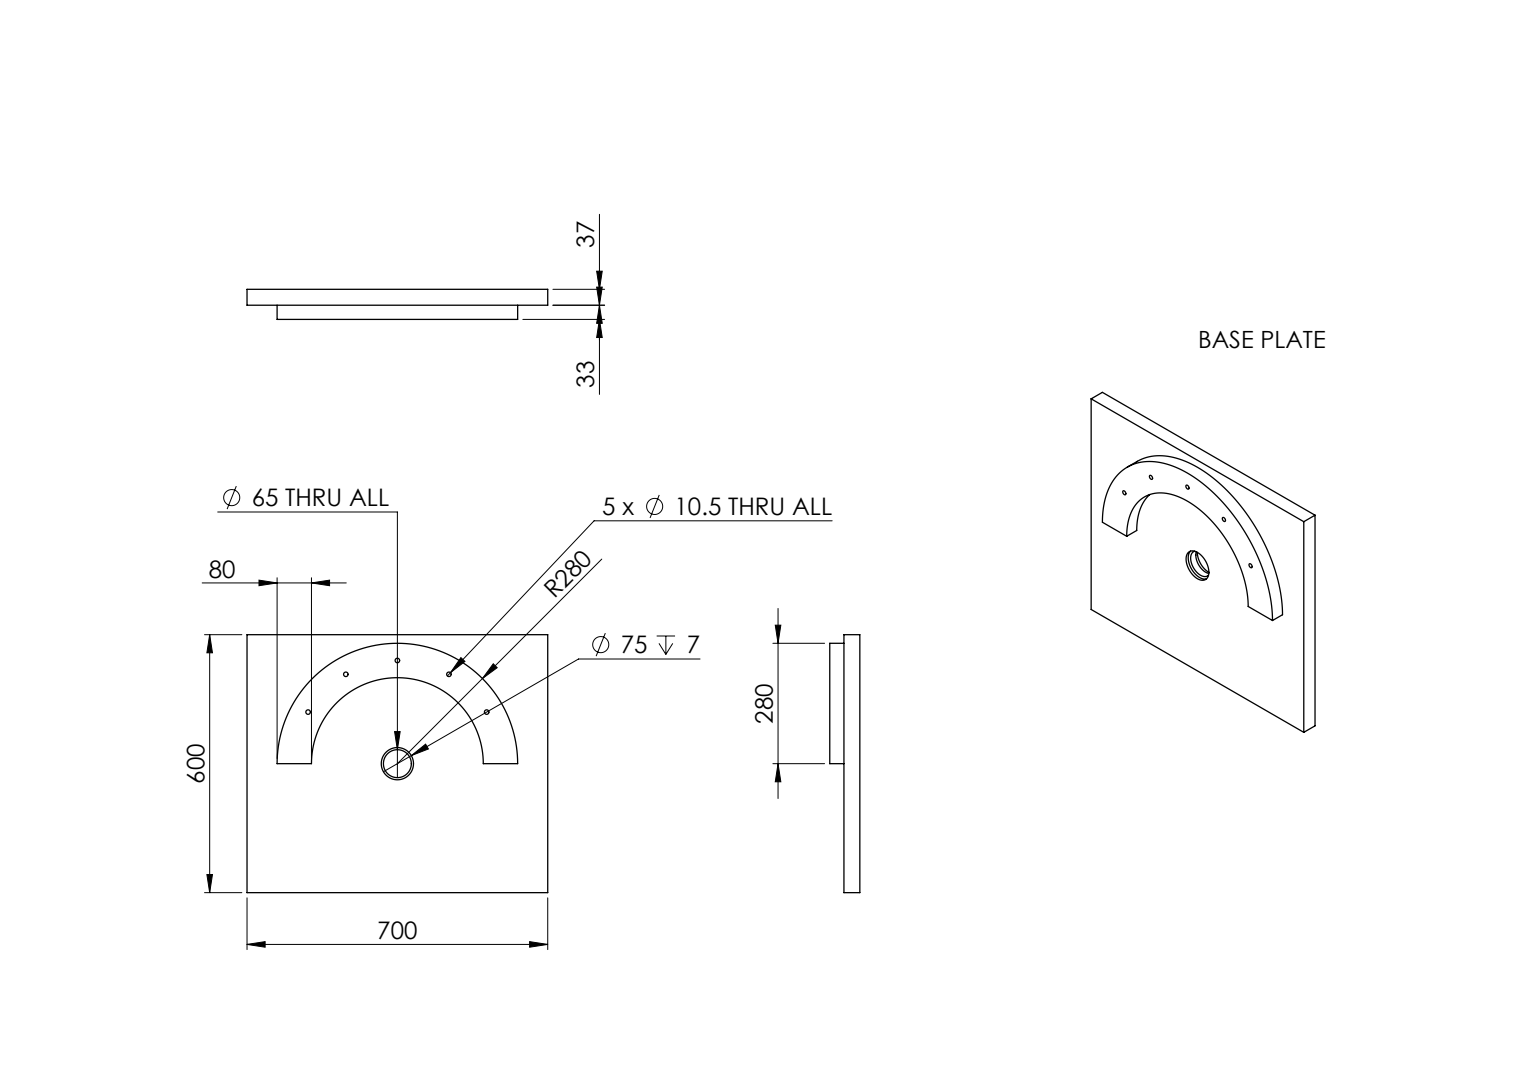
ISO-10303-21;
HEADER;
FILE_DESCRIPTION (('STEP AP214'),
    '1' );
FILE_NAME ('base plate.step',
    '2026-10-23T05:12:30',
    ( '' ),
    ( '' ),
    'SwSTEP 2.0',
    'SolidWorks 2026',
    '' );
FILE_SCHEMA (( 'AUTOMOTIVE_DESIGN' ));
ENDSEC;

DATA;
#3=SURFACE_STYLE_USAGE ( .BOTH. , #3079 ) ;
#17=DIRECTION ( 'NONE',  ( 1.000000000000000000, 0.000000000000000000, 0.000000000000000000 ) ) ;
#19=FACE_OUTER_BOUND ( 'NONE', #6377, .T. ) ;
#26=DIRECTION ( 'NONE',  ( -0.000000000000000000, -0.000000000000000000, 1.000000000000000000 ) ) ;
#42=ORIENTED_EDGE ( 'NONE', *, *, #2330, .T. ) ;
#45=AXIS2_PLACEMENT_3D ( 'NONE', #3946, #5204, #2688 ) ;
#49=ORIENTED_EDGE ( 'NONE', *, *, #2998, .F. ) ;
#51=DIRECTION ( 'NONE',  ( -0.000000000000000000, -0.000000000000000000, 1.000000000000000000 ) ) ;
#61=MECHANICAL_DESIGN_GEOMETRIC_PRESENTATION_REPRESENTATION('',(#4091),#6487);
#62=FACE_BOUND ( 'NONE', #7747, .T. ) ;
#67=DIRECTION ( 'NONE',  ( -0.000000000000000000, 0.000000000000000000, 1.000000000000000000 ) ) ;
#76=SURFACE_STYLE_FILL_AREA ( #5998 ) ;
#98=AXIS2_PLACEMENT_3D ( 'NONE', #4234, #3767, #1954 ) ;
#99=DIRECTION ( 'NONE',  ( 0.000000000000000000, 0.000000000000000000, 1.000000000000000000 ) ) ;
#107=ORIENTED_EDGE ( 'NONE', *, *, #1973, .T. ) ;
#109=ORIENTED_EDGE ( 'NONE', *, *, #3940, .F. ) ;
#123=DIRECTION ( 'NONE',  ( 1.000000000000000000, 0.000000000000000000, 0.000000000000000000 ) ) ;
#128=EDGE_CURVE ( 'NONE', #1948, #4169, #2830, .T. ) ;
#130=ORIENTED_EDGE ( 'NONE', *, *, #1178, .T. ) ;
#144=FACE_OUTER_BOUND ( 'NONE', #3867, .T. ) ;
#154=VERTEX_POINT ( 'NONE', #7084 ) ;
#160=DIRECTION ( 'NONE',  ( 1.000000000000000000, 0.000000000000000000, 0.000000000000000000 ) ) ;
#166=DIRECTION ( 'NONE',  ( -1.000000000000000000, 0.000000000000000000, 0.000000000000000000 ) ) ;
#182=FACE_OUTER_BOUND ( 'NONE', #3425, .T. ) ;
#185=VERTEX_POINT ( 'NONE', #2518 ) ;
#206=EDGE_LOOP ( 'NONE', ( #7630, #2753 ) ) ;
#208=FACE_OUTER_BOUND ( 'NONE', #6661, .T. ) ;
#217=ORIENTED_EDGE ( 'NONE', *, *, #263, .T. ) ;
#218=EDGE_CURVE ( 'NONE', #491, #1814, #4911, .T. ) ;
#245=CARTESIAN_POINT ( 'NONE',  ( 207.8429183184021269, 119.9981648402868331, -50.00000000000000000 ) ) ;
#253=FACE_OUTER_BOUND ( 'NONE', #5709, .T. ) ;
#257=VERTEX_POINT ( 'NONE', #4355 ) ;
#263=EDGE_CURVE ( 'NONE', #257, #1814, #3618, .T. ) ;
#265=ORIENTED_EDGE ( 'NONE', *, *, #789, .F. ) ;
#269=FACE_OUTER_BOUND ( 'NONE', #4910, .T. ) ;
#275=LINE ( 'NONE', #5724, #2339 ) ;
#329=LINE ( 'NONE', #3997, #6288 ) ;
#335=ORIENTED_EDGE ( 'NONE', *, *, #1569, .F. ) ;
#366=DIRECTION ( 'NONE',  ( 1.000000000000000000, 0.000000000000000000, 0.000000000000000000 ) ) ;
#376=LINE ( 'NONE', #524, #671 ) ;
#377=CARTESIAN_POINT ( 'NONE',  ( 199.9963296805737230, -4.796075449120964792E-12, -50.00000000000004263 ) ) ;
#390=LINE ( 'NONE', #2812, #6033 ) ;
#396=( NAMED_UNIT ( * ) PLANE_ANGLE_UNIT ( ) SI_UNIT ( $, .RADIAN. ) );
#399=ADVANCED_FACE ( 'NONE', ( #917 ), #3849, .F. ) ;
#403=DIRECTION ( 'NONE',  ( -1.000000000000000000, 0.000000000000000000, 0.000000000000000000 ) ) ;
#404=ORIENTED_EDGE ( 'NONE', *, *, #2745, .T. ) ;
#413=CARTESIAN_POINT ( 'NONE',  ( -279.9963296805736945, 3.428966089163216048E-14, 576.0908266162076643 ) ) ;
#416=DIRECTION ( 'NONE',  ( -0.000000000000000000, -0.000000000000000000, 1.000000000000000000 ) ) ;
#422=VECTOR ( 'NONE', #416, 1000.000000000000000 ) ;
#433=CONICAL_SURFACE ( 'NONE', #5480, 37.49999999999997868, 1.029744258676654090 ) ;
#441=CARTESIAN_POINT ( 'NONE',  ( 0.000000000000000000, 0.000000000000000000, -112.9999999999999716 ) ) ;
#468=AXIS2_PLACEMENT_3D ( 'NONE', #1319, #7361, #6181 ) ;
#470=EDGE_CURVE ( 'NONE', #491, #1561, #4433, .T. ) ;
#486=CARTESIAN_POINT ( 'NONE',  ( -350.0000000000000000, 300.0000000000001137, -120.0000000000000000 ) ) ;
#488=DIRECTION ( 'NONE',  ( -1.000000000000000000, 0.000000000000000000, 0.000000000000000000 ) ) ;
#491=VERTEX_POINT ( 'NONE', #486 ) ;
#501=CIRCLE ( 'NONE', #6302, 279.9963296805736945 ) ;
#506=FACE_OUTER_BOUND ( 'NONE', #4471, .T. ) ;
#513=FACE_OUTER_BOUND ( 'NONE', #3270, .T. ) ;
#524=CARTESIAN_POINT ( 'NONE',  ( -1.852913429038039572, -299.9999999999999432, -120.0000000000000000 ) ) ;
#525=MANIFOLD_SOLID_BREP ( 'M10 Clearance Hole1', #6120 ) ;
#548=CARTESIAN_POINT ( 'NONE',  ( 350.0000000000000000, 37.15382499588017140, -1041.954445729288636 ) ) ;
#567=APPLICATION_CONTEXT ( 'automotive_design' ) ;
#569=DIRECTION ( 'NONE',  ( 1.000000000000000000, -1.586032892321652729E-16, 0.000000000000000000 ) ) ;
#575=DIRECTION ( 'NONE',  ( 1.000000000000000000, 0.000000000000000000, 0.000000000000000000 ) ) ;
#586=ORIENTED_EDGE ( 'NONE', *, *, #1973, .F. ) ;
#588=CIRCLE ( 'NONE', #4736, 5.249999999999991118 ) ;
#592=CARTESIAN_POINT ( 'NONE',  ( -279.9963296805736945, 3.428966089163216048E-14, -82.99999999999998579 ) ) ;
#604=DIRECTION ( 'NONE',  ( -0.000000000000000000, -0.000000000000000000, -1.000000000000000000 ) ) ;
#607=CARTESIAN_POINT ( 'NONE',  ( 0.000000000000000000, 0.000000000000000000, -50.00000000000000000 ) ) ;
#618=FACE_OUTER_BOUND ( 'NONE', #3198, .T. ) ;
#621=DIRECTION ( 'NONE',  ( 1.000000000000000000, -1.586032892321652729E-16, 0.000000000000000000 ) ) ;
#632=EDGE_CURVE ( 'NONE', #7413, #257, #5381, .T. ) ;
#638=CARTESIAN_POINT ( 'NONE',  ( -199.9963296805737230, 2.449248649845333917E-14, -82.99999999999998579 ) ) ;
#639=FACE_OUTER_BOUND ( 'NONE', #3468, .T. ) ;
#652=FACE_BOUND ( 'NONE', #7710, .T. ) ;
#657=CARTESIAN_POINT ( 'NONE',  ( 37.49999999999997868, 4.592425496802572000E-15, -112.9999999999999716 ) ) ;
#658=ADVANCED_FACE ( 'NONE', ( #4193 ), #3609, .F. ) ;
#668=EDGE_CURVE ( 'NONE', #3544, #1948, #6635, .T. ) ;
#669=VERTEX_POINT ( 'NONE', #3097 ) ;
#671=VECTOR ( 'NONE', #569, 1000.000000000000000 ) ;
#684=DIRECTION ( 'NONE',  ( -0.000000000000000000, 0.000000000000000000, -1.000000000000000000 ) ) ;
#701=ORIENTED_EDGE ( 'NONE', *, *, #2330, .F. ) ;
#703=CARTESIAN_POINT ( 'NONE',  ( 37.49999999999997868, 4.592425496802572000E-15, -119.9999999999999858 ) ) ;
#704=ADVANCED_FACE ( 'NONE', ( #6716 ), #7273, .F. ) ;
#718=CIRCLE ( 'NONE', #468, 5.250000000000004441 ) ;
#734=CARTESIAN_POINT ( 'NONE',  ( -114.7481648402875578, 207.8429183184017859, -50.00000000000000000 ) ) ;
#739=DIRECTION ( 'NONE',  ( -0.000000000000000000, -0.000000000000000000, -1.000000000000000000 ) ) ;
#744=ORIENTED_EDGE ( 'NONE', *, *, #4992, .F. ) ;
#746=VERTEX_POINT ( 'NONE', #907 ) ;
#758=CARTESIAN_POINT ( 'NONE',  ( 0.000000000000000000, 0.000000000000000000, -50.00000000000004263 ) ) ;
#763=EDGE_LOOP ( 'NONE', ( #3582, #5792, #5209, #744 ) ) ;
#764=ADVANCED_FACE ( 'NONE', ( #6171 ), #6323, .F. ) ;
#789=EDGE_CURVE ( 'NONE', #4399, #185, #6381, .T. ) ;
#798=ADVANCED_FACE ( 'NONE', ( #4978 ), #2695, .T. ) ;
#803=EDGE_CURVE ( 'NONE', #1238, #1502, #588, .T. ) ;
#816=VERTEX_POINT ( 'NONE', #6283 ) ;
#829=LINE ( 'NONE', #5048, #4387 ) ;
#833=AXIS2_PLACEMENT_3D ( 'NONE', #7236, #1838, #4860 ) ;
#835=DIRECTION ( 'NONE',  ( -0.8571673007021121116, 0.000000000000000000, -0.5150380749100544886 ) ) ;
#839=AXIS2_PLACEMENT_3D ( 'NONE', #2155, #4033, #5889 ) ;
#840=DIRECTION ( 'NONE',  ( 1.000000000000000000, 0.000000000000000000, 0.000000000000000000 ) ) ;
#847=DIRECTION ( 'NONE',  ( 1.000000000000000000, 0.000000000000000000, 0.000000000000000000 ) ) ;
#849=ORIENTED_EDGE ( 'NONE', *, *, #1091, .F. ) ;
#854=CARTESIAN_POINT ( 'NONE',  ( 279.9963296805736945, -6.714540835673234486E-12, -82.99999999999998579 ) ) ;
#855=CARTESIAN_POINT ( 'NONE',  ( 0.000000000000000000, 0.000000000000000000, -119.9999999999999858 ) ) ;
#874=ORIENTED_EDGE ( 'NONE', *, *, #1580, .T. ) ;
#875=DIRECTION ( 'NONE',  ( -0.000000000000000000, -0.000000000000000000, 1.000000000000000000 ) ) ;
#884=ORIENTED_EDGE ( 'NONE', *, *, #2648, .F. ) ;
#885=ORIENTED_EDGE ( 'NONE', *, *, #632, .F. ) ;
#890=ADVANCED_FACE ( 'NONE', ( #513 ), #3951, .F. ) ;
#899=ORIENTED_EDGE ( 'NONE', *, *, #4517, .T. ) ;
#907=CARTESIAN_POINT ( 'NONE',  ( 114.7481648402866625, 207.8429183184022122, -120.0000000000000000 ) ) ;
#912=DIRECTION ( 'NONE',  ( -0.000000000000000000, -0.000000000000000000, 1.000000000000000000 ) ) ;
#917=FACE_OUTER_BOUND ( 'NONE', #7070, .T. ) ;
#925=ORIENTED_EDGE ( 'NONE', *, *, #1091, .T. ) ;
#932=CARTESIAN_POINT ( 'NONE',  ( 199.9963296805737230, -4.796075449120964792E-12, -50.00000000000004263 ) ) ;
#933=ORIENTED_EDGE ( 'NONE', *, *, #2159, .T. ) ;
#936=ORIENTED_EDGE ( 'NONE', *, *, #5900, .T. ) ;
#946=EDGE_CURVE ( 'NONE', #2474, #3424, #4485, .T. ) ;
#951=FACE_OUTER_BOUND ( 'NONE', #7184, .T. ) ;
#957=DIRECTION ( 'NONE',  ( 0.000000000000000000, 0.000000000000000000, 1.000000000000000000 ) ) ;
#961=ORIENTED_EDGE ( 'NONE', *, *, #1772, .T. ) ;
#962=EDGE_LOOP ( 'NONE', ( #3910, #335 ) ) ;
#968=FACE_OUTER_BOUND ( 'NONE', #763, .T. ) ;
#970=AXIS2_PLACEMENT_3D ( 'NONE', #3411, #7665, #488 ) ;
#998=DIRECTION ( 'NONE',  ( -0.000000000000000000, -0.000000000000000000, -1.000000000000000000 ) ) ;
#1000=ORIENTED_EDGE ( 'NONE', *, *, #5715, .F. ) ;
#1021=LINE ( 'NONE', #1705, #4153 ) ;
#1025=VERTEX_POINT ( 'NONE', #7652 ) ;
#1036=CARTESIAN_POINT ( 'NONE',  ( -350.0000000000000000, 300.0000000000001137, -82.99999999999998579 ) ) ;
#1046=DIRECTION ( 'NONE',  ( -0.000000000000000000, -0.000000000000000000, 1.000000000000000000 ) ) ;
#1053=VERTEX_POINT ( 'NONE', #5653 ) ;
#1056=ORIENTED_EDGE ( 'NONE', *, *, #7068, .F. ) ;
#1073=( GEOMETRIC_REPRESENTATION_CONTEXT ( 3 ) GLOBAL_UNCERTAINTY_ASSIGNED_CONTEXT ( ( #4788 ) ) GLOBAL_UNIT_ASSIGNED_CONTEXT ( ( #5810, #396, #4629 ) ) REPRESENTATION_CONTEXT ( 'NONE', 'WORKASPACE' ) );
#1082=ORIENTED_EDGE ( 'NONE', *, *, #1569, .T. ) ;
#1086=CIRCLE ( 'NONE', #2109, 37.49999999999997868 ) ;
#1091=EDGE_CURVE ( 'NONE', #5886, #6942, #3740, .T. ) ;
#1099=LINE ( 'NONE', #1749, #2193 ) ;
#1104=ADVANCED_FACE ( 'NONE', ( #208 ), #3770, .F. ) ;
#1121=VERTEX_POINT ( 'NONE', #2665 ) ;
#1123=AXIS2_PLACEMENT_3D ( 'NONE', #6696, #67, #6816 ) ;
#1135=DIRECTION ( 'NONE',  ( -1.000000000000000000, 1.586032892321652729E-16, 0.000000000000000000 ) ) ;
#1138=EDGE_CURVE ( 'NONE', #3181, #5886, #1999, .T. ) ;
#1153=CARTESIAN_POINT ( 'NONE',  ( -37.49999999999997868, 4.592425496802572000E-15, -90.00000000000000000 ) ) ;
#1161=EDGE_LOOP ( 'NONE', ( #2545, #5550, #1660, #6503 ) ) ;
#1164=PLANE ( 'NONE',  #6663 ) ;
#1171=ORIENTED_EDGE ( 'NONE', *, *, #4898, .F. ) ;
#1178=EDGE_CURVE ( 'NONE', #4200, #3050, #4365, .T. ) ;
#1185=CARTESIAN_POINT ( 'NONE',  ( 0.000000000000000000, 0.000000000000000000, -82.99999999999998579 ) ) ;
#1191=VERTEX_POINT ( 'NONE', #2121 ) ;
#1198=CARTESIAN_POINT ( 'NONE',  ( 0.000000000000000000, 0.000000000000000000, -109.9956969048621716 ) ) ;
#1221=ORIENTED_EDGE ( 'NONE', *, *, #7269, .F. ) ;
#1231=DIRECTION ( 'NONE',  ( 0.000000000000000000, 1.000000000000000000, 0.000000000000000000 ) ) ;
#1236=EDGE_CURVE ( 'NONE', #2058, #5637, #1988, .T. ) ;
#1238=VERTEX_POINT ( 'NONE', #2857 ) ;
#1242=ADVANCED_FACE ( 'NONE', ( #1631 ), #5932, .T. ) ;
#1264=DIRECTION ( 'NONE',  ( -1.000000000000000000, 2.398081733190337496E-14, 0.000000000000000000 ) ) ;
#1272=PLANE ( 'NONE',  #4013 ) ;
#1291=ORIENTED_EDGE ( 'NONE', *, *, #4755, .T. ) ;
#1294=FILL_AREA_STYLE_COLOUR ( '', #5225 ) ;
#1301=CARTESIAN_POINT ( 'NONE',  ( 0.000000000000000000, 0.000000000000000000, 0.000000000000000000 ) ) ;
#1311=CYLINDRICAL_SURFACE ( 'NONE', #45, 5.249999999999991118 ) ;
#1316=ORIENTED_EDGE ( 'NONE', *, *, #218, .F. ) ;
#1317=CARTESIAN_POINT ( 'NONE',  ( -350.0000000000000000, 300.0000000000001137, -1041.954445729288636 ) ) ;
#1319=CARTESIAN_POINT ( 'NONE',  ( 207.8429183184021269, 119.9981648402868331, -50.00000000000000000 ) ) ;
#1333=ADVANCED_FACE ( 'NONE', ( #3407 ), #2862, .F. ) ;
#1335=VERTEX_POINT ( 'NONE', #6368 ) ;
#1336=AXIS2_PLACEMENT_3D ( 'NONE', #5762, #5167, #4621 ) ;
#1345=CIRCLE ( 'NONE', #2867, 5.249999999999991118 ) ;
#1348=CARTESIAN_POINT ( 'NONE',  ( 0.000000000000000000, 0.000000000000000000, -90.00000000000000000 ) ) ;
#1354=DIRECTION ( 'NONE',  ( 1.000000000000000000, 0.000000000000000000, 0.000000000000000000 ) ) ;
#1358=CARTESIAN_POINT ( 'NONE',  ( -125.2481648402875578, 207.8429183184017859, -50.00000000000000000 ) ) ;
#1364=AXIS2_PLACEMENT_3D ( 'NONE', #4356, #3812, #6774 ) ;
#1372=EDGE_CURVE ( 'NONE', #6339, #1121, #4871, .T. ) ;
#1374=UNCERTAINTY_MEASURE_WITH_UNIT (LENGTH_MEASURE( 1.000000000000000082E-05 ), #4771, 'distance_accuracy_value', 'NONE');
#1380=EDGE_CURVE ( 'NONE', #1191, #2413, #1086, .T. ) ;
#1389=CARTESIAN_POINT ( 'NONE',  ( 37.49999999999997868, 0.000000000000000000, -82.99999999999998579 ) ) ;
#1391=CARTESIAN_POINT ( 'NONE',  ( 125.2481648402866199, 207.8429183184022122, -50.00000000000000000 ) ) ;
#1394=CARTESIAN_POINT ( 'NONE',  ( 0.000000000000000000, 0.000000000000000000, -109.9956969048621716 ) ) ;
#1427=EDGE_CURVE ( 'NONE', #1502, #1238, #1345, .T. ) ;
#1432=DIRECTION ( 'NONE',  ( 0.000000000000000000, -1.000000000000000000, 0.000000000000000000 ) ) ;
#1435=DIRECTION ( 'NONE',  ( 1.000000000000000000, 0.000000000000000000, 0.000000000000000000 ) ) ;
#1437=AXIS2_PLACEMENT_3D ( 'NONE', #4551, #6220, #1517 ) ;
#1439=CARTESIAN_POINT ( 'NONE',  ( 0.000000000000000000, 0.000000000000000000, -82.99999999999998579 ) ) ;
#1444=CIRCLE ( 'NONE', #5855, 5.249999999999976907 ) ;
#1462=CARTESIAN_POINT ( 'NONE',  ( -5.134781488891348999E-13, 239.9963296805737230, -50.00000000000000000 ) ) ;
#1471=AXIS2_PLACEMENT_3D ( 'NONE', #5311, #1685, #2953 ) ;
#1477=DIRECTION ( 'NONE',  ( -0.000000000000000000, -0.000000000000000000, -1.000000000000000000 ) ) ;
#1480=EDGE_CURVE ( 'NONE', #4264, #669, #7752, .T. ) ;
#1494=AXIS2_PLACEMENT_3D ( 'NONE', #7712, #1046, #2332 ) ;
#1502=VERTEX_POINT ( 'NONE', #1358 ) ;
#1515=CARTESIAN_POINT ( 'NONE',  ( 37.49999999999997868, 0.000000000000000000, -90.00000000000000000 ) ) ;
#1517=DIRECTION ( 'NONE',  ( 1.000000000000000000, 0.000000000000000000, 0.000000000000000000 ) ) ;
#1540=VERTEX_POINT ( 'NONE', #2563 ) ;
#1561=VERTEX_POINT ( 'NONE', #4319 ) ;
#1563=CARTESIAN_POINT ( 'NONE',  ( 199.9963296805737230, -4.796075449120964792E-12, 576.0908266162076643 ) ) ;
#1569=EDGE_CURVE ( 'NONE', #5426, #1540, #718, .T. ) ;
#1570=AXIS2_PLACEMENT_3D ( 'NONE', #3623, #6029, #621 ) ;
#1580=EDGE_CURVE ( 'NONE', #2827, #7413, #3032, .T. ) ;
#1581=DIRECTION ( 'NONE',  ( 1.000000000000000000, 0.000000000000000000, 0.000000000000000000 ) ) ;
#1590=ORIENTED_EDGE ( 'NONE', *, *, #5900, .F. ) ;
#1602=AXIS2_PLACEMENT_3D ( 'NONE', #4476, #7433, #1435 ) ;
#1614=LINE ( 'NONE', #2260, #7101 ) ;
#1620=ADVANCED_FACE ( 'NONE', ( #6812 ), #2247, .F. ) ;
#1631=FACE_OUTER_BOUND ( 'NONE', #3790, .T. ) ;
#1649=CARTESIAN_POINT ( 'NONE',  ( -119.9981648402875578, 207.8429183184017859, -120.0000000000000000 ) ) ;
#1650=EDGE_LOOP ( 'NONE', ( #6505, #6800, #3164, #3817 ) ) ;
#1653=EDGE_LOOP ( 'NONE', ( #4040, #404, #1082, #1782 ) ) ;
#1660=ORIENTED_EDGE ( 'NONE', *, *, #5572, .T. ) ;
#1666=AXIS2_PLACEMENT_3D ( 'NONE', #2734, #5765, #3954 ) ;
#1677=EDGE_CURVE ( 'NONE', #5637, #7551, #3223, .T. ) ;
#1685=DIRECTION ( 'NONE',  ( -0.000000000000000000, -0.000000000000000000, 1.000000000000000000 ) ) ;
#1698=PLANE ( 'NONE',  #2023 ) ;
#1705=CARTESIAN_POINT ( 'NONE',  ( 213.0929183184020985, 119.9981648402868331, -50.00000000000000000 ) ) ;
#1730=VECTOR ( 'NONE', #6808, 1000.000000000000000 ) ;
#1749=CARTESIAN_POINT ( 'NONE',  ( -350.0000000000000000, 37.15382499588017140, -82.99999999999998579 ) ) ;
#1753=FACE_OUTER_BOUND ( 'NONE', #2499, .T. ) ;
#1757=ORIENTED_EDGE ( 'NONE', *, *, #3553, .T. ) ;
#1758=ORIENTED_EDGE ( 'NONE', *, *, #1677, .F. ) ;
#1759=AXIS2_PLACEMENT_3D ( 'NONE', #3147, #6140, #7751 ) ;
#1772=EDGE_CURVE ( 'NONE', #154, #5402, #5005, .T. ) ;
#1779=EDGE_LOOP ( 'NONE', ( #2401, #4296, #6441, #5600 ) ) ;
#1782=ORIENTED_EDGE ( 'NONE', *, *, #3398, .F. ) ;
#1809=DIRECTION ( 'NONE',  ( 1.000000000000000000, 0.000000000000000000, 0.000000000000000000 ) ) ;
#1814=VERTEX_POINT ( 'NONE', #1036 ) ;
#1823=ORIENTED_EDGE ( 'NONE', *, *, #632, .T. ) ;
#1831=PLANE ( 'NONE',  #3254 ) ;
#1838=DIRECTION ( 'NONE',  ( -0.000000000000000000, -0.000000000000000000, -1.000000000000000000 ) ) ;
#1840=PLANE ( 'NONE',  #2011 ) ;
#1847=FACE_BOUND ( 'NONE', #2961, .T. ) ;
#1854=VERTEX_POINT ( 'NONE', #4156 ) ;
#1855=AXIS2_PLACEMENT_3D ( 'NONE', #758, #6837, #3764 ) ;
#1856=ORIENTED_EDGE ( 'NONE', *, *, #1236, .T. ) ;
#1857=CARTESIAN_POINT ( 'NONE',  ( 37.49999999999997868, 0.000000000000000000, -82.99999999999998579 ) ) ;
#1858=( NAMED_UNIT ( * ) PLANE_ANGLE_UNIT ( ) SI_UNIT ( $, .RADIAN. ) );
#1863=CARTESIAN_POINT ( 'NONE',  ( 0.000000000000000000, 0.000000000000000000, -90.00000000000000000 ) ) ;
#1873=CARTESIAN_POINT ( 'NONE',  ( -207.8429183184026670, 119.9981648402859378, -50.00000000000000000 ) ) ;
#1876=FACE_BOUND ( 'NONE', #2789, .T. ) ;
#1880=ADVANCED_FACE ( 'NONE', ( #6413 ), #4707, .F. ) ;
#1881=ORIENTED_EDGE ( 'NONE', *, *, #6017, .F. ) ;
#1885=CARTESIAN_POINT ( 'NONE',  ( -1.791896790581761989, 35.93034554373089406, -119.9999999999999858 ) ) ;
#1890=DIRECTION ( 'NONE',  ( 0.8571673007021121116, 1.049727191138618449E-16, -0.5150380749100544886 ) ) ;
#1930=VERTEX_POINT ( 'NONE', #6447 ) ;
#1934=AXIS2_PLACEMENT_3D ( 'NONE', #1946, #5608, #3834 ) ;
#1941=VECTOR ( 'NONE', #7153, 1000.000000000000000 ) ;
#1946=CARTESIAN_POINT ( 'NONE',  ( 0.000000000000000000, 0.000000000000000000, -82.99999999999998579 ) ) ;
#1947=VERTEX_POINT ( 'NONE', #2982 ) ;
#1948=VERTEX_POINT ( 'NONE', #3529 ) ;
#1954=DIRECTION ( 'NONE',  ( 1.000000000000000000, 0.000000000000000000, 0.000000000000000000 ) ) ;
#1963=LINE ( 'NONE', #3887, #5776 ) ;
#1967=PLANE ( 'NONE',  #1570 ) ;
#1973=EDGE_CURVE ( 'NONE', #1053, #1854, #5260, .T. ) ;
#1988=CIRCLE ( 'NONE', #4241, 32.49999999999997158 ) ;
#1993=DIRECTION ( 'NONE',  ( 1.000000000000000000, 0.000000000000000000, 0.000000000000000000 ) ) ;
#1999=LINE ( 'NONE', #3182, #1730 ) ;
#2003=CARTESIAN_POINT ( 'NONE',  ( -1.852913429038039572, -299.9999999999999432, -82.99999999999998579 ) ) ;
#2007=ORIENTED_EDGE ( 'NONE', *, *, #1480, .T. ) ;
#2011=AXIS2_PLACEMENT_3D ( 'NONE', #4904, #3569, #6608 ) ;
#2018=LINE ( 'NONE', #932, #4711 ) ;
#2023=AXIS2_PLACEMENT_3D ( 'NONE', #548, #6550, #6508 ) ;
#2047=CARTESIAN_POINT ( 'NONE',  ( -125.2481648402875578, 207.8429183184017859, -50.00000000000000000 ) ) ;
#2058=VERTEX_POINT ( 'NONE', #6720 ) ;
#2070=DIRECTION ( 'NONE',  ( -0.000000000000000000, -0.000000000000000000, 1.000000000000000000 ) ) ;
#2080=DIRECTION ( 'NONE',  ( -0.000000000000000000, -0.000000000000000000, 1.000000000000000000 ) ) ;
#2090=ORIENTED_EDGE ( 'NONE', *, *, #1427, .T. ) ;
#2109=AXIS2_PLACEMENT_3D ( 'NONE', #4677, #2408, #2333 ) ;
#2121=CARTESIAN_POINT ( 'NONE',  ( -37.49999999999997868, 0.000000000000000000, -119.9999999999999858 ) ) ;
#2124=CARTESIAN_POINT ( 'NONE',  ( -5.134781488891348999E-13, 239.9963296805737230, -50.00000000000000000 ) ) ;
#2126=DIRECTION ( 'NONE',  ( 1.000000000000000000, 0.000000000000000000, 0.000000000000000000 ) ) ;
#2128=DIRECTION ( 'NONE',  ( -0.000000000000000000, -0.000000000000000000, 1.000000000000000000 ) ) ;
#2132=ORIENTED_EDGE ( 'NONE', *, *, #4820, .F. ) ;
#2139=AXIS2_PLACEMENT_3D ( 'NONE', #2521, #4912, #1809 ) ;
#2141=ORIENTED_EDGE ( 'NONE', *, *, #6017, .T. ) ;
#2148=ORIENTED_EDGE ( 'NONE', *, *, #5326, .F. ) ;
#2155=CARTESIAN_POINT ( 'NONE',  ( -350.0000000000000000, 37.15382499588017140, -1041.954445729288636 ) ) ;
#2159=EDGE_CURVE ( 'NONE', #4490, #1053, #6877, .T. ) ;
#2162=DIRECTION ( 'NONE',  ( 1.000000000000000000, 0.000000000000000000, 0.000000000000000000 ) ) ;
#2177=EDGE_LOOP ( 'NONE', ( #874, #1823, #217, #3763 ) ) ;
#2190=CARTESIAN_POINT ( 'NONE',  ( 350.0000000000000000, 300.0000000000000000, -120.0000000000000000 ) ) ;
#2193=VECTOR ( 'NONE', #5322, 1000.000000000000000 ) ;
#2226=CARTESIAN_POINT ( 'NONE',  ( 0.000000000000000000, 0.000000000000000000, -112.9999999999999716 ) ) ;
#2247=CONICAL_SURFACE ( 'NONE', #3120, 37.49999999999997868, 1.029744258676654090 ) ;
#2260=CARTESIAN_POINT ( 'NONE',  ( -202.5929183184026954, 119.9981648402859378, -50.00000000000000000 ) ) ;
#2262=DIRECTION ( 'NONE',  ( -0.000000000000000000, -0.000000000000000000, 1.000000000000000000 ) ) ;
#2263=VERTEX_POINT ( 'NONE', #2893 ) ;
#2271=VECTOR ( 'NONE', #2292, 1000.000000000000000 ) ;
#2292=DIRECTION ( 'NONE',  ( -0.000000000000000000, -0.000000000000000000, 1.000000000000000000 ) ) ;
#2310=LINE ( 'NONE', #7146, #3009 ) ;
#2330=EDGE_CURVE ( 'NONE', #1561, #2827, #390, .T. ) ;
#2332=DIRECTION ( 'NONE',  ( 1.000000000000000000, 0.000000000000000000, 0.000000000000000000 ) ) ;
#2333=DIRECTION ( 'NONE',  ( -1.000000000000000000, 0.000000000000000000, 0.000000000000000000 ) ) ;
#2339=VECTOR ( 'NONE', #835, 1000.000000000000000 ) ;
#2343=( LENGTH_UNIT ( ) NAMED_UNIT ( * ) SI_UNIT ( .MILLI., .METRE. ) );
#2347=CARTESIAN_POINT ( 'NONE',  ( -37.49999999999997868, 0.000000000000000000, -112.9999999999999716 ) ) ;
#2364=PRODUCT_DEFINITION_CONTEXT ( 'detailed design', #5505, 'design' ) ;
#2400=EDGE_CURVE ( 'NONE', #5402, #1121, #2310, .T. ) ;
#2401=ORIENTED_EDGE ( 'NONE', *, *, #7219, .F. ) ;
#2404=CIRCLE ( 'NONE', #3275, 279.9963296805736945 ) ;
#2408=DIRECTION ( 'NONE',  ( -0.000000000000000000, -0.000000000000000000, -1.000000000000000000 ) ) ;
#2413=VERTEX_POINT ( 'NONE', #4581 ) ;
#2420=SHAPE_REPRESENTATION_RELATIONSHIP ( 'NONE' , 'NONE' ,  #5012, #4435 ) ;
#2426=ADVANCED_FACE ( 'NONE', ( #639 ), #1831, .F. ) ;
#2427=DIRECTION ( 'NONE',  ( 1.000000000000000000, 0.000000000000000000, 0.000000000000000000 ) ) ;
#2429=DIRECTION ( 'NONE',  ( -0.000000000000000000, -0.000000000000000000, 1.000000000000000000 ) ) ;
#2432=CARTESIAN_POINT ( 'NONE',  ( 350.0000000000000000, 37.15382499588017140, -82.99999999999998579 ) ) ;
#2434=DIRECTION ( 'NONE',  ( -0.000000000000000000, -0.000000000000000000, -1.000000000000000000 ) ) ;
#2451=EDGE_LOOP ( 'NONE', ( #4442, #7521, #3780, #6080 ) ) ;
#2457=CARTESIAN_POINT ( 'NONE',  ( 5.249999999999474198, 239.9963296805737230, -120.0000000000000000 ) ) ;
#2460=CARTESIAN_POINT ( 'NONE',  ( -213.0929183184026670, 119.9981648402859378, -120.0000000000000000 ) ) ;
#2474=VERTEX_POINT ( 'NONE', #4777 ) ;
#2490=LINE ( 'NONE', #734, #2950 ) ;
#2499=EDGE_LOOP ( 'NONE', ( #1000, #2624, #6856, #3389 ) ) ;
#2510=DIRECTION ( 'NONE',  ( -1.000000000000000000, 0.000000000000000000, 0.000000000000000000 ) ) ;
#2517=CIRCLE ( 'NONE', #2139, 5.249999999999976907 ) ;
#2518=CARTESIAN_POINT ( 'NONE',  ( -199.9963296805737230, 2.449248649845333917E-14, -50.00000000000004263 ) ) ;
#2521=CARTESIAN_POINT ( 'NONE',  ( 207.8429183184021269, 119.9981648402868331, -120.0000000000000000 ) ) ;
#2527=AXIS2_PLACEMENT_3D ( 'NONE', #5547, #2564, #7365 ) ;
#2532=AXIS2_PLACEMENT_3D ( 'NONE', #7104, #5966, #6004 ) ;
#2544=FACE_OUTER_BOUND ( 'NONE', #1161, .T. ) ;
#2545=ORIENTED_EDGE ( 'NONE', *, *, #4371, .F. ) ;
#2553=EDGE_CURVE ( 'NONE', #746, #4490, #2626, .T. ) ;
#2563=CARTESIAN_POINT ( 'NONE',  ( 213.0929183184021269, 119.9981648402868331, -50.00000000000000000 ) ) ;
#2564=DIRECTION ( 'NONE',  ( -0.000000000000000000, -0.000000000000000000, 1.000000000000000000 ) ) ;
#2565=LINE ( 'NONE', #657, #6215 ) ;
#2576=ORIENTED_EDGE ( 'NONE', *, *, #5572, .F. ) ;
#2588=ORIENTED_EDGE ( 'NONE', *, *, #218, .T. ) ;
#2591=CARTESIAN_POINT ( 'NONE',  ( -5.134781488891348999E-13, 239.9963296805737230, -50.00000000000000000 ) ) ;
#2593=CARTESIAN_POINT ( 'NONE',  ( -350.0000000000000000, 37.15382499588017140, -120.0000000000000000 ) ) ;
#2603=ORIENTED_EDGE ( 'NONE', *, *, #4568, .F. ) ;
#2607=CARTESIAN_POINT ( 'NONE',  ( 32.49999999999997158, 3.980102097228894682E-15, -109.9956969048621716 ) ) ;
#2617=ORIENTED_EDGE ( 'NONE', *, *, #1372, .T. ) ;
#2624=ORIENTED_EDGE ( 'NONE', *, *, #3553, .F. ) ;
#2626=CIRCLE ( 'NONE', #2749, 5.249999999999976907 ) ;
#2644=DIRECTION ( 'NONE',  ( -0.000000000000000000, -0.000000000000000000, 1.000000000000000000 ) ) ;
#2648=EDGE_CURVE ( 'NONE', #2058, #3050, #829, .T. ) ;
#2656=AXIS2_PLACEMENT_3D ( 'NONE', #1863, #4813, #2427 ) ;
#2665=CARTESIAN_POINT ( 'NONE',  ( -213.0929183184026954, 119.9981648402859378, -50.00000000000000000 ) ) ;
#2688=DIRECTION ( 'NONE',  ( 1.000000000000000000, 0.000000000000000000, 0.000000000000000000 ) ) ;
#2695=CYLINDRICAL_SURFACE ( 'NONE', #7136, 279.9963296805736945 ) ;
#2697=VECTOR ( 'NONE', #7686, 1000.000000000000000 ) ;
#2702=DIRECTION ( 'NONE',  ( -0.000000000000000000, -0.000000000000000000, -1.000000000000000000 ) ) ;
#2710=CARTESIAN_POINT ( 'NONE',  ( 0.000000000000000000, 0.000000000000000000, -93.00430309513780003 ) ) ;
#2718=CARTESIAN_POINT ( 'NONE',  ( -5.134781488891348999E-13, 239.9963296805737230, -50.00000000000000000 ) ) ;
#2725=DIRECTION ( 'NONE',  ( -0.000000000000000000, -0.000000000000000000, -1.000000000000000000 ) ) ;
#2726=AXIS2_PLACEMENT_3D ( 'NONE', #5685, #6763, #166 ) ;
#2734=CARTESIAN_POINT ( 'NONE',  ( -207.8429183184026670, 119.9981648402859378, -50.00000000000000000 ) ) ;
#2745=EDGE_CURVE ( 'NONE', #1930, #5426, #7677, .T. ) ;
#2749=AXIS2_PLACEMENT_3D ( 'NONE', #6123, #3130, #123 ) ;
#2751=ORIENTED_EDGE ( 'NONE', *, *, #1427, .F. ) ;
#2753=ORIENTED_EDGE ( 'NONE', *, *, #6264, .F. ) ;
#2755=CARTESIAN_POINT ( 'NONE',  ( -279.9963296805736945, 3.428966089163216048E-14, -50.00000000000004263 ) ) ;
#2761=CIRCLE ( 'NONE', #1494, 5.249999999999987566 ) ;
#2762=ORIENTED_EDGE ( 'NONE', *, *, #5185, .F. ) ;
#2776=ORIENTED_EDGE ( 'NONE', *, *, #4898, .T. ) ;
#2779=CIRCLE ( 'NONE', #4792, 5.250000000000004441 ) ;
#2789=EDGE_LOOP ( 'NONE', ( #849, #2576 ) ) ;
#2790=ORIENTED_EDGE ( 'NONE', *, *, #1380, .F. ) ;
#2792=EDGE_CURVE ( 'NONE', #5001, #6427, #6671, .T. ) ;
#2800=ORIENTED_EDGE ( 'NONE', *, *, #4755, .F. ) ;
#2804=AXIS2_PLACEMENT_3D ( 'NONE', #7498, #912, #3179 ) ;
#2812=CARTESIAN_POINT ( 'NONE',  ( -350.0000000000000000, -299.9999999999998863, -1041.954445729288636 ) ) ;
#2813=VECTOR ( 'NONE', #604, 1000.000000000000000 ) ;
#2826=AXIS2_PLACEMENT_3D ( 'NONE', #1348, #6053, #5494 ) ;
#2827=VERTEX_POINT ( 'NONE', #6579 ) ;
#2830=LINE ( 'NONE', #4675, #6755 ) ;
#2855=ORIENTED_EDGE ( 'NONE', *, *, #7451, .F. ) ;
#2857=CARTESIAN_POINT ( 'NONE',  ( -114.7481648402875578, 207.8429183184017859, -50.00000000000000000 ) ) ;
#2862=CONICAL_SURFACE ( 'NONE', #3869, 37.49999999999997868, 1.029744258676654090 ) ;
#2863=FACE_OUTER_BOUND ( 'NONE', #5939, .T. ) ;
#2867=AXIS2_PLACEMENT_3D ( 'NONE', #2912, #7129, #7049 ) ;
#2877=ORIENTED_EDGE ( 'NONE', *, *, #3649, .T. ) ;
#2878=ORIENTED_EDGE ( 'NONE', *, *, #6636, .T. ) ;
#2882=ADVANCED_FACE ( 'NONE', ( #6658, #4916, #6104 ), #6778, .T. ) ;
#2891=DIRECTION ( 'NONE',  ( -0.000000000000000000, -0.000000000000000000, -1.000000000000000000 ) ) ;
#2893=CARTESIAN_POINT ( 'NONE',  ( -5.250000000000500933, 239.9963296805737230, -120.0000000000000000 ) ) ;
#2908=CIRCLE ( 'NONE', #2656, 37.49999999999997868 ) ;
#2909=EDGE_LOOP ( 'NONE', ( #4888, #3977 ) ) ;
#2912=CARTESIAN_POINT ( 'NONE',  ( -119.9981648402875578, 207.8429183184017859, -50.00000000000000000 ) ) ;
#2914=VECTOR ( 'NONE', #1135, 1000.000000000000000 ) ;
#2937=ORIENTED_EDGE ( 'NONE', *, *, #4071, .F. ) ;
#2950=VECTOR ( 'NONE', #4917, 1000.000000000000000 ) ;
#2953=DIRECTION ( 'NONE',  ( 1.000000000000000000, 0.000000000000000000, 0.000000000000000000 ) ) ;
#2961=EDGE_LOOP ( 'NONE', ( #6146, #3172 ) ) ;
#2967=ORIENTED_EDGE ( 'NONE', *, *, #6359, .T. ) ;
#2973=CARTESIAN_POINT ( 'NONE',  ( 207.8429183184021269, 119.9981648402868331, -50.00000000000000000 ) ) ;
#2977=ORIENTED_EDGE ( 'NONE', *, *, #4424, .F. ) ;
#2978=STYLED_ITEM('',(#7809),#525);
#2982=CARTESIAN_POINT ( 'NONE',  ( -37.49999999999997868, 4.592425496802572000E-15, -90.00000000000000000 ) ) ;
#2994=DIRECTION ( 'NONE',  ( -0.9987587364483917485, -0.04980950078059114688, 0.000000000000000000 ) ) ;
#2998=EDGE_CURVE ( 'NONE', #6427, #5001, #5917, .T. ) ;
#3006=CARTESIAN_POINT ( 'NONE',  ( -279.9963296805736945, 3.428966089163216048E-14, -50.00000000000004263 ) ) ;
#3009=VECTOR ( 'NONE', #5214, 1000.000000000000000 ) ;
#3016=VECTOR ( 'NONE', #5734, 1000.000000000000000 ) ;
#3026=EDGE_CURVE ( 'NONE', #4169, #669, #2404, .T. ) ;
#3028=EDGE_CURVE ( 'NONE', #5001, #1502, #3262, .T. ) ;
#3030=EDGE_CURVE ( 'NONE', #7307, #6615, #7423, .T. ) ;
#3031=CYLINDRICAL_SURFACE ( 'NONE', #1759, 5.249999999999991118 ) ;
#3032=LINE ( 'NONE', #2003, #5257 ) ;
#3040=ADVANCED_FACE ( 'NONE', ( #253 ), #5031, .F. ) ;
#3050=VERTEX_POINT ( 'NONE', #4729 ) ;
#3064=PRODUCT_DEFINITION_FORMATION_WITH_SPECIFIED_SOURCE ( 'ANY', '', #3721, .NOT_KNOWN. ) ;
#3066=FACE_BOUND ( 'NONE', #2909, .T. ) ;
#3072=ORIENTED_EDGE ( 'NONE', *, *, #6264, .T. ) ;
#3079=SURFACE_SIDE_STYLE ('',( #76 ) ) ;
#3097=CARTESIAN_POINT ( 'NONE',  ( -279.9963296805736945, 3.428966089163216048E-14, -82.99999999999998579 ) ) ;
#3101=CARTESIAN_POINT ( 'NONE',  ( 0.000000000000000000, 0.000000000000000000, -90.00000000000000000 ) ) ;
#3120=AXIS2_PLACEMENT_3D ( 'NONE', #6027, #26, #2126 ) ;
#3130=DIRECTION ( 'NONE',  ( -0.000000000000000000, -0.000000000000000000, 1.000000000000000000 ) ) ;
#3135=ORIENTED_EDGE ( 'NONE', *, *, #3030, .F. ) ;
#3136=DIRECTION ( 'NONE',  ( -0.000000000000000000, -0.000000000000000000, 1.000000000000000000 ) ) ;
#3141=ADVANCED_FACE ( 'NONE', ( #506 ), #1698, .T. ) ;
#3147=CARTESIAN_POINT ( 'NONE',  ( -119.9981648402875578, 207.8429183184017859, -50.00000000000000000 ) ) ;
#3162=ORIENTED_EDGE ( 'NONE', *, *, #3406, .T. ) ;
#3164=ORIENTED_EDGE ( 'NONE', *, *, #4992, .T. ) ;
#3172=ORIENTED_EDGE ( 'NONE', *, *, #4371, .T. ) ;
#3179=DIRECTION ( 'NONE',  ( 1.000000000000000000, 0.000000000000000000, 0.000000000000000000 ) ) ;
#3181=VERTEX_POINT ( 'NONE', #2457 ) ;
#3182=CARTESIAN_POINT ( 'NONE',  ( 5.249999999999477751, 239.9963296805737230, -50.00000000000000000 ) ) ;
#3198=EDGE_LOOP ( 'NONE', ( #4699, #49, #3545, #6273 ) ) ;
#3205=CYLINDRICAL_SURFACE ( 'NONE', #5829, 5.249999999999992006 ) ;
#3223=LINE ( 'NONE', #1515, #4499 ) ;
#3225=PRODUCT_DEFINITION_SHAPE ( 'NONE', 'NONE',  #6722 ) ;
#3244=DIRECTION ( 'NONE',  ( -0.000000000000000000, -0.000000000000000000, 1.000000000000000000 ) ) ;
#3254=AXIS2_PLACEMENT_3D ( 'NONE', #4930, #4341, #1264 ) ;
#3261=EDGE_CURVE ( 'NONE', #4264, #816, #501, .T. ) ;
#3262=LINE ( 'NONE', #2047, #6922 ) ;
#3267=ORIENTED_EDGE ( 'NONE', *, *, #2553, .T. ) ;
#3270=EDGE_LOOP ( 'NONE', ( #2132, #3416, #2007, #3573 ) ) ;
#3275=AXIS2_PLACEMENT_3D ( 'NONE', #6853, #3856, #7437 ) ;
#3286=CARTESIAN_POINT ( 'NONE',  ( -119.9981648402875578, 207.8429183184017859, -50.00000000000000000 ) ) ;
#3298=CARTESIAN_POINT ( 'NONE',  ( 5.249999999999482192, 239.9963296805737230, -50.00000000000000000 ) ) ;
#3305=DIRECTION ( 'NONE',  ( -0.000000000000000000, -0.000000000000000000, -1.000000000000000000 ) ) ;
#3313=AXIS2_PLACEMENT_3D ( 'NONE', #2973, #2429, #6710 ) ;
#3322=DIRECTION ( 'NONE',  ( -0.000000000000000000, -0.000000000000000000, 1.000000000000000000 ) ) ;
#3326=ADVANCED_FACE ( 'NONE', ( #968 ), #3385, .F. ) ;
#3333=LINE ( 'NONE', #6446, #3016 ) ;
#3361=AXIS2_PLACEMENT_3D ( 'NONE', #1394, #2702, #5101 ) ;
#3385=CYLINDRICAL_SURFACE ( 'NONE', #3905, 37.49999999999997868 ) ;
#3389=ORIENTED_EDGE ( 'NONE', *, *, #3030, .T. ) ;
#3398=EDGE_CURVE ( 'NONE', #1025, #1540, #1021, .T. ) ;
#3403=EDGE_CURVE ( 'NONE', #3181, #2263, #4408, .T. ) ;
#3406=EDGE_CURVE ( 'NONE', #5637, #4200, #6557, .T. ) ;
#3407=FACE_OUTER_BOUND ( 'NONE', #5112, .T. ) ;
#3411=CARTESIAN_POINT ( 'NONE',  ( 0.000000000000000000, 0.000000000000000000, 576.0908266162076643 ) ) ;
#3416=ORIENTED_EDGE ( 'NONE', *, *, #5302, .T. ) ;
#3417=ORIENTED_EDGE ( 'NONE', *, *, #2400, .F. ) ;
#3424=VERTEX_POINT ( 'NONE', #2347 ) ;
#3425=EDGE_LOOP ( 'NONE', ( #7709, #6522, #933, #107 ) ) ;
#3435=CARTESIAN_POINT ( 'NONE',  ( 32.49999999999997158, 3.980102097228894682E-15, -119.9999999999999858 ) ) ;
#3449=CARTESIAN_POINT ( 'NONE',  ( 350.0000000000000000, -300.0000000000000000, -1041.954445729288636 ) ) ;
#3455=ADVANCED_FACE ( 'NONE', ( #1753 ), #7188, .F. ) ;
#3464=CONICAL_SURFACE ( 'NONE', #4846, 37.49999999999997868, 1.029744258676654090 ) ;
#3468=EDGE_LOOP ( 'NONE', ( #2603, #6699, #6821, #3583 ) ) ;
#3479=MECHANICAL_DESIGN_GEOMETRIC_PRESENTATION_REPRESENTATION('',(#2978),#1073);
#3496=DIRECTION ( 'NONE',  ( 1.000000000000000000, -2.398081733190337496E-14, 0.000000000000000000 ) ) ;
#3529=CARTESIAN_POINT ( 'NONE',  ( 199.9963296805737230, -4.796075449120964792E-12, -82.99999999999998579 ) ) ;
#3542=DIRECTION ( 'NONE',  ( -0.000000000000000000, -0.000000000000000000, 1.000000000000000000 ) ) ;
#3544=VERTEX_POINT ( 'NONE', #638 ) ;
#3545=ORIENTED_EDGE ( 'NONE', *, *, #7068, .T. ) ;
#3553=EDGE_CURVE ( 'NONE', #7551, #1947, #2908, .T. ) ;
#3569=DIRECTION ( 'NONE',  ( 1.586032892321652729E-16, 1.000000000000000000, -0.000000000000000000 ) ) ;
#3573=ORIENTED_EDGE ( 'NONE', *, *, #5287, .T. ) ;
#3582=ORIENTED_EDGE ( 'NONE', *, *, #946, .F. ) ;
#3583=ORIENTED_EDGE ( 'NONE', *, *, #128, .T. ) ;
#3586=ORIENTED_EDGE ( 'NONE', *, *, #7544, .F. ) ;
#3589=LINE ( 'NONE', #592, #5207 ) ;
#3609=CYLINDRICAL_SURFACE ( 'NONE', #4359, 5.249999999999976907 ) ;
#3618=LINE ( 'NONE', #7281, #5174 ) ;
#3623=CARTESIAN_POINT ( 'NONE',  ( -1.852913429038039572, -299.9999999999999432, -1041.954445729288636 ) ) ;
#3649=EDGE_CURVE ( 'NONE', #1854, #1053, #2779, .T. ) ;
#3654=FACE_BOUND ( 'NONE', #7069, .T. ) ;
#3663=ORIENTED_EDGE ( 'NONE', *, *, #7331, .F. ) ;
#3680=DIRECTION ( 'NONE',  ( -0.000000000000000000, -0.000000000000000000, -1.000000000000000000 ) ) ;
#3712=ORIENTED_EDGE ( 'NONE', *, *, #2553, .F. ) ;
#3721=PRODUCT ( 'base plate', 'base plate', '', ( #6142 ) ) ;
#3740=CIRCLE ( 'NONE', #7390, 5.249999999999995559 ) ;
#3758=DIRECTION ( 'NONE',  ( 0.000000000000000000, 0.000000000000000000, 1.000000000000000000 ) ) ;
#3763=ORIENTED_EDGE ( 'NONE', *, *, #5185, .T. ) ;
#3764=DIRECTION ( 'NONE',  ( -1.000000000000000000, 8.881784197001252323E-16, 0.000000000000000000 ) ) ;
#3767=DIRECTION ( 'NONE',  ( -0.000000000000000000, -0.000000000000000000, 1.000000000000000000 ) ) ;
#3768=CARTESIAN_POINT ( 'NONE',  ( -114.7481648402875578, 207.8429183184017859, -120.0000000000000000 ) ) ;
#3770=CYLINDRICAL_SURFACE ( 'NONE', #5119, 5.249999999999976907 ) ;
#3779=AXIS2_PLACEMENT_3D ( 'NONE', #1649, #3542, #6457 ) ;
#3780=ORIENTED_EDGE ( 'NONE', *, *, #3026, .F. ) ;
#3790=EDGE_LOOP ( 'NONE', ( #1316, #5982, #42, #2762 ) ) ;
#3791=AXIS2_PLACEMENT_3D ( 'NONE', #1185, #5253, #5329 ) ;
#3812=DIRECTION ( 'NONE',  ( -0.000000000000000000, -0.000000000000000000, -1.000000000000000000 ) ) ;
#3817=ORIENTED_EDGE ( 'NONE', *, *, #1380, .T. ) ;
#3834=DIRECTION ( 'NONE',  ( 1.000000000000000000, 0.000000000000000000, 0.000000000000000000 ) ) ;
#3839=LINE ( 'NONE', #6914, #5974 ) ;
#3849=CYLINDRICAL_SURFACE ( 'NONE', #3861, 37.49999999999997868 ) ;
#3856=DIRECTION ( 'NONE',  ( 0.000000000000000000, 0.000000000000000000, 1.000000000000000000 ) ) ;
#3861=AXIS2_PLACEMENT_3D ( 'NONE', #7431, #2080, #4510 ) ;
#3867=EDGE_LOOP ( 'NONE', ( #701, #4554, #2141, #7439 ) ) ;
#3869=AXIS2_PLACEMENT_3D ( 'NONE', #441, #4108, #3958 ) ;
#3875=DIRECTION ( 'NONE',  ( -0.000000000000000000, -0.000000000000000000, -1.000000000000000000 ) ) ;
#3887=CARTESIAN_POINT ( 'NONE',  ( 279.9963296805736945, -6.714540835673234486E-12, 576.0908266162076643 ) ) ;
#3905=AXIS2_PLACEMENT_3D ( 'NONE', #855, #3305, #6935 ) ;
#3910=ORIENTED_EDGE ( 'NONE', *, *, #6636, .F. ) ;
#3936=AXIS2_PLACEMENT_3D ( 'NONE', #6326, #6842, #7388 ) ;
#3940=EDGE_CURVE ( 'NONE', #6520, #491, #5318, .T. ) ;
#3943=AXIS2_PLACEMENT_3D ( 'NONE', #4689, #2262, #1581 ) ;
#3946=CARTESIAN_POINT ( 'NONE',  ( -119.9981648402875578, 207.8429183184017859, -50.00000000000000000 ) ) ;
#3948=CIRCLE ( 'NONE', #6091, 37.49999999999997868 ) ;
#3951=PLANE ( 'NONE',  #1336 ) ;
#3954=DIRECTION ( 'NONE',  ( 1.000000000000000000, 0.000000000000000000, 0.000000000000000000 ) ) ;
#3957=AXIS2_PLACEMENT_3D ( 'NONE', #5803, #3322, #6875 ) ;
#3958=DIRECTION ( 'NONE',  ( -1.000000000000000000, 0.000000000000000000, 0.000000000000000000 ) ) ;
#3967=EDGE_LOOP ( 'NONE', ( #5256, #4298, #6212, #1758 ) ) ;
#3969=LINE ( 'NONE', #1563, #2813 ) ;
#3977=ORIENTED_EDGE ( 'NONE', *, *, #2792, .T. ) ;
#3997=CARTESIAN_POINT ( 'NONE',  ( 350.0000000000000000, 300.0000000000000000, -1041.954445729288636 ) ) ;
#4012=ORIENTED_EDGE ( 'NONE', *, *, #6127, .T. ) ;
#4013=AXIS2_PLACEMENT_3D ( 'NONE', #607, #684, #7314 ) ;
#4020=EDGE_CURVE ( 'NONE', #2474, #2413, #7215, .T. ) ;
#4033=DIRECTION ( 'NONE',  ( -1.000000000000000000, 0.000000000000000000, 0.000000000000000000 ) ) ;
#4040=ORIENTED_EDGE ( 'NONE', *, *, #4517, .F. ) ;
#4064=CYLINDRICAL_SURFACE ( 'NONE', #1666, 5.249999999999976907 ) ;
#4071=EDGE_CURVE ( 'NONE', #7551, #7307, #4923, .T. ) ;
#4091=STYLED_ITEM ( 'NONE', ( #7297 ), #4435 ) ;
#4101=DIRECTION ( 'NONE',  ( -0.000000000000000000, -0.000000000000000000, -1.000000000000000000 ) ) ;
#4108=DIRECTION ( 'NONE',  ( -0.000000000000000000, -0.000000000000000000, -1.000000000000000000 ) ) ;
#4114=VECTOR ( 'NONE', #6576, 1000.000000000000000 ) ;
#4119=VECTOR ( 'NONE', #5649, 1000.000000000000000 ) ;
#4134=DIRECTION ( 'NONE',  ( -0.000000000000000000, -0.000000000000000000, -1.000000000000000000 ) ) ;
#4135=( NAMED_UNIT ( * ) PLANE_ANGLE_UNIT ( ) SI_UNIT ( $, .RADIAN. ) );
#4150=EDGE_LOOP ( 'NONE', ( #3417, #5360, #7292, #2617 ) ) ;
#4153=VECTOR ( 'NONE', #4735, 1000.000000000000000 ) ;
#4155=CARTESIAN_POINT ( 'NONE',  ( -125.2481648402875578, 207.8429183184017859, -120.0000000000000000 ) ) ;
#4156=CARTESIAN_POINT ( 'NONE',  ( 114.7481648402866341, 207.8429183184022122, -50.00000000000000000 ) ) ;
#4169=VERTEX_POINT ( 'NONE', #854 ) ;
#4185=VECTOR ( 'NONE', #99, 1000.000000000000000 ) ;
#4190=DIRECTION ( 'NONE',  ( -0.000000000000000000, -0.000000000000000000, 1.000000000000000000 ) ) ;
#4193=FACE_OUTER_BOUND ( 'NONE', #1653, .T. ) ;
#4199=DIRECTION ( 'NONE',  ( -0.000000000000000000, -0.000000000000000000, 1.000000000000000000 ) ) ;
#4200=VERTEX_POINT ( 'NONE', #2607 ) ;
#4234=CARTESIAN_POINT ( 'NONE',  ( 119.9981648402866341, 207.8429183184022122, -50.00000000000000000 ) ) ;
#4237=FACE_OUTER_BOUND ( 'NONE', #7378, .T. ) ;
#4241=AXIS2_PLACEMENT_3D ( 'NONE', #4665, #7577, #7661 ) ;
#4242=DIRECTION ( 'NONE',  ( -0.000000000000000000, -0.000000000000000000, 1.000000000000000000 ) ) ;
#4252=DIRECTION ( 'NONE',  ( -0.000000000000000000, -0.000000000000000000, 1.000000000000000000 ) ) ;
#4256=EDGE_LOOP ( 'NONE', ( #3712, #4782, #2877, #4791 ) ) ;
#4264=VERTEX_POINT ( 'NONE', #2755 ) ;
#4267=DIRECTION ( 'NONE',  ( 1.000000000000000000, 0.000000000000000000, 0.000000000000000000 ) ) ;
#4269=FACE_BOUND ( 'NONE', #962, .T. ) ;
#4296=ORIENTED_EDGE ( 'NONE', *, *, #789, .T. ) ;
#4298=ORIENTED_EDGE ( 'NONE', *, *, #7269, .T. ) ;
#4309=CIRCLE ( 'NONE', #3936, 5.249999999999976907 ) ;
#4319=CARTESIAN_POINT ( 'NONE',  ( -350.0000000000000000, -299.9999999999998863, -120.0000000000000000 ) ) ;
#4334=AXIS2_PLACEMENT_3D ( 'NONE', #2718, #2644, #6825 ) ;
#4338=CARTESIAN_POINT ( 'NONE',  ( 119.9981648402866341, 207.8429183184022122, -50.00000000000000000 ) ) ;
#4340=VECTOR ( 'NONE', #7667, 1000.000000000000000 ) ;
#4341=DIRECTION ( 'NONE',  ( 2.398081733190337496E-14, 1.000000000000000000, -0.000000000000000000 ) ) ;
#4355=CARTESIAN_POINT ( 'NONE',  ( 350.0000000000000000, 300.0000000000000000, -82.99999999999998579 ) ) ;
#4356=CARTESIAN_POINT ( 'NONE',  ( 0.000000000000000000, 0.000000000000000000, -119.9999999999999858 ) ) ;
#4358=SHAPE_DEFINITION_REPRESENTATION ( #3225, #5012 ) ;
#4359=AXIS2_PLACEMENT_3D ( 'NONE', #5421, #51, #17 ) ;
#4365=CIRCLE ( 'NONE', #3361, 32.49999999999997158 ) ;
#4371=EDGE_CURVE ( 'NONE', #2263, #3181, #2761, .T. ) ;
#4376=UNCERTAINTY_MEASURE_WITH_UNIT (LENGTH_MEASURE( 1.000000000000000082E-05 ), #2343, 'distance_accuracy_value', 'NONE');
#4387=VECTOR ( 'NONE', #7011, 1000.000000000000000 ) ;
#4389=CARTESIAN_POINT ( 'NONE',  ( 350.0000000000000000, 37.15382499588017140, -120.0000000000000000 ) ) ;
#4399=VERTEX_POINT ( 'NONE', #377 ) ;
#4408=CIRCLE ( 'NONE', #2532, 5.249999999999987566 ) ;
#4424=EDGE_CURVE ( 'NONE', #2263, #6942, #6066, .T. ) ;
#4433=LINE ( 'NONE', #2593, #7496 ) ;
#4435=ADVANCED_BREP_SHAPE_REPRESENTATION ( '', ( #525, #7485 ), #4585 ) ;
#4440=DIRECTION ( 'NONE',  ( -0.000000000000000000, -0.000000000000000000, 1.000000000000000000 ) ) ;
#4441=ORIENTED_EDGE ( 'NONE', *, *, #3026, .T. ) ;
#4442=ORIENTED_EDGE ( 'NONE', *, *, #668, .F. ) ;
#4448=DIRECTION ( 'NONE',  ( -1.000000000000000000, 0.000000000000000000, 0.000000000000000000 ) ) ;
#4451=DIRECTION ( 'NONE',  ( -1.000000000000000000, 2.398081733190337496E-14, 0.000000000000000000 ) ) ;
#4468=DIRECTION ( 'NONE',  ( -0.000000000000000000, 1.000000000000000000, 0.000000000000000000 ) ) ;
#4471=EDGE_LOOP ( 'NONE', ( #1881, #6947, #1291, #885 ) ) ;
#4476=CARTESIAN_POINT ( 'NONE',  ( -207.8429183184026670, 119.9981648402859378, -120.0000000000000000 ) ) ;
#4483=ADVANCED_FACE ( 'NONE', ( #652, #3654, #1847, #3066, #5465, #62, #7283 ), #1164, .T. ) ;
#4485=CIRCLE ( 'NONE', #4495, 37.49999999999997868 ) ;
#4490=VERTEX_POINT ( 'NONE', #7325 ) ;
#4495=AXIS2_PLACEMENT_3D ( 'NONE', #6436, #2891, #7103 ) ;
#4499=VECTOR ( 'NONE', #5063, 1000.000000000000000 ) ;
#4501=CARTESIAN_POINT ( 'NONE',  ( 0.000000000000000000, 0.000000000000000000, 576.0908266162076643 ) ) ;
#4508=DIRECTION ( 'NONE',  ( -0.000000000000000000, -0.000000000000000000, 1.000000000000000000 ) ) ;
#4510=DIRECTION ( 'NONE',  ( 1.000000000000000000, 0.000000000000000000, 0.000000000000000000 ) ) ;
#4517=EDGE_CURVE ( 'NONE', #1930, #1025, #2517, .T. ) ;
#4518=CYLINDRICAL_SURFACE ( 'NONE', #1437, 5.249999999999976907 ) ;
#4528=CARTESIAN_POINT ( 'NONE',  ( 32.49999999999997158, 3.980102097228894682E-15, -93.00430309513780003 ) ) ;
#4541=VECTOR ( 'NONE', #739, 1000.000000000000000 ) ;
#4551=CARTESIAN_POINT ( 'NONE',  ( 119.9981648402866341, 207.8429183184022122, -50.00000000000000000 ) ) ;
#4554=ORIENTED_EDGE ( 'NONE', *, *, #7187, .T. ) ;
#4555=ADVANCED_FACE ( 'NONE', ( #618 ), #3031, .F. ) ;
#4558=VECTOR ( 'NONE', #4468, 1000.000000000000000 ) ;
#4567=FACE_OUTER_BOUND ( 'NONE', #5780, .T. ) ;
#4568=EDGE_CURVE ( 'NONE', #816, #4169, #1963, .T. ) ;
#4581=CARTESIAN_POINT ( 'NONE',  ( 37.49999999999997868, 4.592425496802572000E-15, -119.9999999999999858 ) ) ;
#4583=ORIENTED_EDGE ( 'NONE', *, *, #3403, .F. ) ;
#4585=( GEOMETRIC_REPRESENTATION_CONTEXT ( 3 ) GLOBAL_UNCERTAINTY_ASSIGNED_CONTEXT ( ( #4376 ) ) GLOBAL_UNIT_ASSIGNED_CONTEXT ( ( #2343, #4135, #5955 ) ) REPRESENTATION_CONTEXT ( 'NONE', 'WORKASPACE' ) );
#4593=LINE ( 'NONE', #3449, #4340 ) ;
#4617=ADVANCED_FACE ( 'NONE', ( #6180 ), #6293, .F. ) ;
#4621=DIRECTION ( 'NONE',  ( -1.000000000000000000, 1.224646799147352961E-16, 0.000000000000000000 ) ) ;
#4629=( NAMED_UNIT ( * ) SI_UNIT ( $, .STERADIAN. ) SOLID_ANGLE_UNIT ( ) );
#4665=CARTESIAN_POINT ( 'NONE',  ( 0.000000000000000000, 0.000000000000000000, -93.00430309513780003 ) ) ;
#4675=CARTESIAN_POINT ( 'NONE',  ( 199.9963296805737230, -4.796075449120964792E-12, -82.99999999999998579 ) ) ;
#4677=CARTESIAN_POINT ( 'NONE',  ( 0.000000000000000000, 0.000000000000000000, -119.9999999999999858 ) ) ;
#4689=CARTESIAN_POINT ( 'NONE',  ( 119.9981648402866341, 207.8429183184022122, -50.00000000000000000 ) ) ;
#4699=ORIENTED_EDGE ( 'NONE', *, *, #3028, .F. ) ;
#4707=CYLINDRICAL_SURFACE ( 'NONE', #970, 199.9963296805737230 ) ;
#4711=VECTOR ( 'NONE', #4451, 1000.000000000000000 ) ;
#4715=ORIENTED_EDGE ( 'NONE', *, *, #2792, .F. ) ;
#4729=CARTESIAN_POINT ( 'NONE',  ( -32.49999999999997158, 0.000000000000000000, -109.9956969048621716 ) ) ;
#4735=DIRECTION ( 'NONE',  ( -0.000000000000000000, -0.000000000000000000, 1.000000000000000000 ) ) ;
#4736=AXIS2_PLACEMENT_3D ( 'NONE', #3286, #2070, #1993 ) ;
#4743=EDGE_LOOP ( 'NONE', ( #586, #7748 ) ) ;
#4755=EDGE_CURVE ( 'NONE', #6520, #257, #329, .T. ) ;
#4767=ORIENTED_EDGE ( 'NONE', *, *, #1178, .F. ) ;
#4771=( LENGTH_UNIT ( ) NAMED_UNIT ( * ) SI_UNIT ( .MILLI., .METRE. ) );
#4774=ORIENTED_EDGE ( 'NONE', *, *, #5086, .T. ) ;
#4777=CARTESIAN_POINT ( 'NONE',  ( 37.49999999999997868, 4.592425496802572000E-15, -112.9999999999999716 ) ) ;
#4782=ORIENTED_EDGE ( 'NONE', *, *, #7584, .T. ) ;
#4786=LINE ( 'NONE', #5423, #5783 ) ;
#4788=UNCERTAINTY_MEASURE_WITH_UNIT (LENGTH_MEASURE( 1.000000000000000082E-05 ), #5810, 'distance_accuracy_value', 'NONE');
#4789=DIRECTION ( 'NONE',  ( 1.000000000000000000, 0.000000000000000000, 0.000000000000000000 ) ) ;
#4791=ORIENTED_EDGE ( 'NONE', *, *, #2159, .F. ) ;
#4792=AXIS2_PLACEMENT_3D ( 'NONE', #4338, #6756, #160 ) ;
#4813=DIRECTION ( 'NONE',  ( -0.000000000000000000, -0.000000000000000000, 1.000000000000000000 ) ) ;
#4820=EDGE_CURVE ( 'NONE', #185, #3544, #3333, .T. ) ;
#4821=ORIENTED_EDGE ( 'NONE', *, *, #5302, .F. ) ;
#4846=AXIS2_PLACEMENT_3D ( 'NONE', #5347, #998, #403 ) ;
#4860=DIRECTION ( 'NONE',  ( 1.000000000000000000, 0.000000000000000000, 0.000000000000000000 ) ) ;
#4866=CARTESIAN_POINT ( 'NONE',  ( 119.9981648402866341, 207.8429183184022122, -120.0000000000000000 ) ) ;
#4871=CIRCLE ( 'NONE', #1471, 5.250000000000004441 ) ;
#4886=CARTESIAN_POINT ( 'NONE',  ( 202.5929183184021269, 119.9981648402868331, -50.00000000000000000 ) ) ;
#4888=ORIENTED_EDGE ( 'NONE', *, *, #2998, .T. ) ;
#4898=EDGE_CURVE ( 'NONE', #3050, #4200, #6414, .T. ) ;
#4900=ADVANCED_FACE ( 'NONE', ( #4269, #7198, #1876, #6682, #6092, #4567 ), #1272, .F. ) ;
#4904=CARTESIAN_POINT ( 'NONE',  ( -1.852913429037944315, 300.0000000000000568, -1041.954445729288636 ) ) ;
#4910=EDGE_LOOP ( 'NONE', ( #4715, #7484, #2090, #1056 ) ) ;
#4911=LINE ( 'NONE', #1317, #4185 ) ;
#4912=DIRECTION ( 'NONE',  ( -0.000000000000000000, -0.000000000000000000, 1.000000000000000000 ) ) ;
#4916=FACE_BOUND ( 'NONE', #4958, .T. ) ;
#4917=DIRECTION ( 'NONE',  ( -0.000000000000000000, -0.000000000000000000, 1.000000000000000000 ) ) ;
#4923=LINE ( 'NONE', #1857, #6438 ) ;
#4930=CARTESIAN_POINT ( 'NONE',  ( 199.9963296805737230, -4.796075449120964792E-12, 576.0908266162076643 ) ) ;
#4931=DIRECTION ( 'NONE',  ( 1.000000000000000000, 0.000000000000000000, 0.000000000000000000 ) ) ;
#4938=DIRECTION ( 'NONE',  ( -1.000000000000000000, 0.000000000000000000, 0.000000000000000000 ) ) ;
#4958=EDGE_LOOP ( 'NONE', ( #3135, #5897 ) ) ;
#4974=ORIENTED_EDGE ( 'NONE', *, *, #3940, .T. ) ;
#4978=FACE_OUTER_BOUND ( 'NONE', #5833, .T. ) ;
#4992=EDGE_CURVE ( 'NONE', #3424, #1191, #4786, .T. ) ;
#4997=ADVANCED_FACE ( 'NONE', ( #19 ), #1840, .T. ) ;
#5001=VERTEX_POINT ( 'NONE', #4155 ) ;
#5005=CIRCLE ( 'NONE', #1602, 5.249999999999976907 ) ;
#5012=SHAPE_REPRESENTATION ( 'base plate', ( #7485 ), #4585 ) ;
#5015=ORIENTED_EDGE ( 'NONE', *, *, #3261, .F. ) ;
#5031=CYLINDRICAL_SURFACE ( 'NONE', #6551, 32.49999999999997158 ) ;
#5048=CARTESIAN_POINT ( 'NONE',  ( -32.49999999999997158, 0.000000000000000000, -119.9999999999999858 ) ) ;
#5056=CARTESIAN_POINT ( 'NONE',  ( -202.5929183184026670, 119.9981648402859378, -50.00000000000000000 ) ) ;
#5063=DIRECTION ( 'NONE',  ( 0.8571673007021121116, 0.000000000000000000, 0.5150380749100544886 ) ) ;
#5086=EDGE_CURVE ( 'NONE', #3424, #2474, #6668, .T. ) ;
#5101=DIRECTION ( 'NONE',  ( -1.000000000000000000, 0.000000000000000000, 0.000000000000000000 ) ) ;
#5112=EDGE_LOOP ( 'NONE', ( #7202, #1171, #5438, #4774 ) ) ;
#5119=AXIS2_PLACEMENT_3D ( 'NONE', #245, #875, #840 ) ;
#5145=ADVANCED_FACE ( 'NONE', ( #269 ), #1311, .F. ) ;
#5146=VECTOR ( 'NONE', #4242, 1000.000000000000000 ) ;
#5152=LINE ( 'NONE', #1153, #1941 ) ;
#5157=ORIENTED_EDGE ( 'NONE', *, *, #1138, .T. ) ;
#5167=DIRECTION ( 'NONE',  ( 1.224646799147352961E-16, 1.000000000000000000, -0.000000000000000000 ) ) ;
#5174=VECTOR ( 'NONE', #6024, 1000.000000000000000 ) ;
#5185=EDGE_CURVE ( 'NONE', #1814, #2827, #1099, .T. ) ;
#5204=DIRECTION ( 'NONE',  ( -0.000000000000000000, -0.000000000000000000, 1.000000000000000000 ) ) ;
#5207=VECTOR ( 'NONE', #7021, 1000.000000000000000 ) ;
#5208=ORIENTED_EDGE ( 'NONE', *, *, #7082, .T. ) ;
#5209=ORIENTED_EDGE ( 'NONE', *, *, #7310, .T. ) ;
#5214=DIRECTION ( 'NONE',  ( -0.000000000000000000, -0.000000000000000000, 1.000000000000000000 ) ) ;
#5218=AXIS2_PLACEMENT_3D ( 'NONE', #2710, #2128, #2162 ) ;
#5225=COLOUR_RGB ( '',0.8941176470588234615, 0.8941176470588234615, 0.8941176470588234615 ) ;
#5246=LINE ( 'NONE', #3006, #2697 ) ;
#5253=DIRECTION ( 'NONE',  ( -0.000000000000000000, -0.000000000000000000, 1.000000000000000000 ) ) ;
#5256=ORIENTED_EDGE ( 'NONE', *, *, #1236, .F. ) ;
#5257=VECTOR ( 'NONE', #7246, 1000.000000000000000 ) ;
#5260=CIRCLE ( 'NONE', #98, 5.250000000000004441 ) ;
#5287=EDGE_CURVE ( 'NONE', #669, #3544, #3589, .T. ) ;
#5302=EDGE_CURVE ( 'NONE', #185, #4264, #5246, .T. ) ;
#5311=CARTESIAN_POINT ( 'NONE',  ( -207.8429183184026670, 119.9981648402859378, -50.00000000000000000 ) ) ;
#5318=LINE ( 'NONE', #5365, #2914 ) ;
#5322=DIRECTION ( 'NONE',  ( 0.000000000000000000, -1.000000000000000000, 0.000000000000000000 ) ) ;
#5324=ORIENTED_EDGE ( 'NONE', *, *, #5538, .F. ) ;
#5326=EDGE_CURVE ( 'NONE', #154, #6339, #1614, .T. ) ;
#5329=DIRECTION ( 'NONE',  ( 1.000000000000000000, 0.000000000000000000, 0.000000000000000000 ) ) ;
#5347=CARTESIAN_POINT ( 'NONE',  ( 0.000000000000000000, 0.000000000000000000, -112.9999999999999716 ) ) ;
#5349=ORIENTED_EDGE ( 'NONE', *, *, #2400, .T. ) ;
#5350=CIRCLE ( 'NONE', #3957, 5.249999999999976907 ) ;
#5360=ORIENTED_EDGE ( 'NONE', *, *, #1772, .F. ) ;
#5365=CARTESIAN_POINT ( 'NONE',  ( -1.852913429037944315, 300.0000000000000568, -120.0000000000000000 ) ) ;
#5381=LINE ( 'NONE', #2432, #6129 ) ;
#5384=DIRECTION ( 'NONE',  ( -0.000000000000000000, -0.000000000000000000, -1.000000000000000000 ) ) ;
#5390=ORIENTED_EDGE ( 'NONE', *, *, #7187, .F. ) ;
#5396=DIRECTION ( 'NONE',  ( -0.000000000000000000, 0.000000000000000000, -1.000000000000000000 ) ) ;
#5402=VERTEX_POINT ( 'NONE', #2460 ) ;
#5421=CARTESIAN_POINT ( 'NONE',  ( 207.8429183184021269, 119.9981648402868331, -50.00000000000000000 ) ) ;
#5423=CARTESIAN_POINT ( 'NONE',  ( -37.49999999999997868, 0.000000000000000000, -119.9999999999999858 ) ) ;
#5426=VERTEX_POINT ( 'NONE', #4886 ) ;
#5438=ORIENTED_EDGE ( 'NONE', *, *, #7451, .T. ) ;
#5465=FACE_BOUND ( 'NONE', #5908, .T. ) ;
#5474=ORIENTED_EDGE ( 'NONE', *, *, #263, .F. ) ;
#5480=AXIS2_PLACEMENT_3D ( 'NONE', #3101, #4199, #575 ) ;
#5483=ORIENTED_EDGE ( 'NONE', *, *, #3406, .F. ) ;
#5494=DIRECTION ( 'NONE',  ( 1.000000000000000000, 0.000000000000000000, 0.000000000000000000 ) ) ;
#5505=APPLICATION_CONTEXT ( 'automotive_design' ) ;
#5538=EDGE_CURVE ( 'NONE', #816, #4399, #2018, .T. ) ;
#5547=CARTESIAN_POINT ( 'NONE',  ( -119.9981648402875578, 207.8429183184017859, -120.0000000000000000 ) ) ;
#5550=ORIENTED_EDGE ( 'NONE', *, *, #4424, .T. ) ;
#5572=EDGE_CURVE ( 'NONE', #6942, #5886, #7730, .T. ) ;
#5578=EDGE_LOOP ( 'NONE', ( #7095, #2751 ) ) ;
#5600=ORIENTED_EDGE ( 'NONE', *, *, #668, .T. ) ;
#5608=DIRECTION ( 'NONE',  ( -0.000000000000000000, -0.000000000000000000, 1.000000000000000000 ) ) ;
#5630=ORIENTED_EDGE ( 'NONE', *, *, #6305, .F. ) ;
#5637=VERTEX_POINT ( 'NONE', #4528 ) ;
#5649=DIRECTION ( 'NONE',  ( -0.000000000000000000, -0.000000000000000000, 1.000000000000000000 ) ) ;
#5653=CARTESIAN_POINT ( 'NONE',  ( 125.2481648402866341, 207.8429183184022122, -50.00000000000000000 ) ) ;
#5660=CARTESIAN_POINT ( 'NONE',  ( 0.000000000000000000, 0.000000000000000000, -119.9999999999999858 ) ) ;
#5685=CARTESIAN_POINT ( 'NONE',  ( 0.000000000000000000, 0.000000000000000000, -119.9999999999999858 ) ) ;
#5701=EDGE_LOOP ( 'NONE', ( #5390, #7005, #109, #5630 ) ) ;
#5709=EDGE_LOOP ( 'NONE', ( #1856, #3162, #130, #884 ) ) ;
#5715=EDGE_CURVE ( 'NONE', #1947, #6615, #5906, .T. ) ;
#5719=CARTESIAN_POINT ( 'NONE',  ( -5.250000000000509814, 239.9963296805737230, -50.00000000000000000 ) ) ;
#5724=CARTESIAN_POINT ( 'NONE',  ( -37.49999999999997868, 0.000000000000000000, -112.9999999999999716 ) ) ;
#5734=DIRECTION ( 'NONE',  ( -0.000000000000000000, -0.000000000000000000, -1.000000000000000000 ) ) ;
#5762=CARTESIAN_POINT ( 'NONE',  ( -279.9963296805736945, 3.428966089163216048E-14, 576.0908266162076643 ) ) ;
#5765=DIRECTION ( 'NONE',  ( -0.000000000000000000, -0.000000000000000000, 1.000000000000000000 ) ) ;
#5772=DIRECTION ( 'NONE',  ( -0.000000000000000000, -0.000000000000000000, 1.000000000000000000 ) ) ;
#5776=VECTOR ( 'NONE', #1477, 1000.000000000000000 ) ;
#5780=EDGE_LOOP ( 'NONE', ( #5324, #5015, #4821, #265 ) ) ;
#5783=VECTOR ( 'NONE', #5384, 1000.000000000000000 ) ;
#5787=CARTESIAN_POINT ( 'NONE',  ( 0.000000000000000000, 0.000000000000000000, -50.00000000000004263 ) ) ;
#5792=ORIENTED_EDGE ( 'NONE', *, *, #4020, .T. ) ;
#5801=ADVANCED_FACE ( 'NONE', ( #144 ), #1967, .T. ) ;
#5803=CARTESIAN_POINT ( 'NONE',  ( -207.8429183184026670, 119.9981648402859378, -120.0000000000000000 ) ) ;
#5810=( LENGTH_UNIT ( ) NAMED_UNIT ( * ) SI_UNIT ( .MILLI., .METRE. ) );
#5827=CARTESIAN_POINT ( 'NONE',  ( -37.49999999999997868, 4.592425496802572000E-15, -82.99999999999998579 ) ) ;
#5829=AXIS2_PLACEMENT_3D ( 'NONE', #1462, #3244, #4931 ) ;
#5833=EDGE_LOOP ( 'NONE', ( #6584, #6964, #6631, #4441 ) ) ;
#5847=ORIENTED_EDGE ( 'NONE', *, *, #2745, .F. ) ;
#5855=AXIS2_PLACEMENT_3D ( 'NONE', #4866, #4190, #4789 ) ;
#5886=VERTEX_POINT ( 'NONE', #3298 ) ;
#5889=DIRECTION ( 'NONE',  ( 0.000000000000000000, 0.000000000000000000, 1.000000000000000000 ) ) ;
#5897=ORIENTED_EDGE ( 'NONE', *, *, #6834, .F. ) ;
#5900=EDGE_CURVE ( 'NONE', #5637, #2058, #7370, .T. ) ;
#5906=LINE ( 'NONE', #5827, #422 ) ;
#5908=EDGE_LOOP ( 'NONE', ( #961, #6008 ) ) ;
#5912=ADVANCED_FACE ( 'NONE', ( #182 ), #4518, .F. ) ;
#5917=CIRCLE ( 'NONE', #2527, 5.249999999999991118 ) ;
#5931=EDGE_LOOP ( 'NONE', ( #5483, #936, #5960, #2776 ) ) ;
#5932=PLANE ( 'NONE',  #839 ) ;
#5939=EDGE_LOOP ( 'NONE', ( #4767, #5208, #7377, #2855 ) ) ;
#5955=( NAMED_UNIT ( * ) SI_UNIT ( $, .STERADIAN. ) SOLID_ANGLE_UNIT ( ) );
#5960=ORIENTED_EDGE ( 'NONE', *, *, #2648, .T. ) ;
#5966=DIRECTION ( 'NONE',  ( -0.000000000000000000, -0.000000000000000000, 1.000000000000000000 ) ) ;
#5969=EDGE_LOOP ( 'NONE', ( #2977, #4583, #5157, #925 ) ) ;
#5974=VECTOR ( 'NONE', #5772, 1000.000000000000000 ) ;
#5977=DIRECTION ( 'NONE',  ( 1.000000000000000000, 0.000000000000000000, 0.000000000000000000 ) ) ;
#5982=ORIENTED_EDGE ( 'NONE', *, *, #470, .T. ) ;
#5998=FILL_AREA_STYLE ('',( #1294 ) ) ;
#6004=DIRECTION ( 'NONE',  ( 1.000000000000000000, 0.000000000000000000, 0.000000000000000000 ) ) ;
#6007=CARTESIAN_POINT ( 'NONE',  ( -37.49999999999997868, 4.592425496802572000E-15, -82.99999999999998579 ) ) ;
#6008=ORIENTED_EDGE ( 'NONE', *, *, #7544, .T. ) ;
#6017=EDGE_CURVE ( 'NONE', #1335, #7413, #4593, .T. ) ;
#6024=DIRECTION ( 'NONE',  ( -1.000000000000000000, 1.586032892321652482E-16, 0.000000000000000000 ) ) ;
#6027=CARTESIAN_POINT ( 'NONE',  ( 0.000000000000000000, 0.000000000000000000, -90.00000000000000000 ) ) ;
#6029=DIRECTION ( 'NONE',  ( -1.586032892321652729E-16, -1.000000000000000000, 0.000000000000000000 ) ) ;
#6033=VECTOR ( 'NONE', #7066, 1000.000000000000000 ) ;
#6041=AXIS2_PLACEMENT_3D ( 'NONE', #1198, #2434, #7275 ) ;
#6053=DIRECTION ( 'NONE',  ( -0.000000000000000000, -0.000000000000000000, 1.000000000000000000 ) ) ;
#6060=ADVANCED_FACE ( 'NONE', ( #2863 ), #3464, .F. ) ;
#6066=LINE ( 'NONE', #7245, #5146 ) ;
#6080=ORIENTED_EDGE ( 'NONE', *, *, #128, .F. ) ;
#6088=ORIENTED_EDGE ( 'NONE', *, *, #3398, .T. ) ;
#6091=AXIS2_PLACEMENT_3D ( 'NONE', #6205, #3680, #2510 ) ;
#6092=FACE_BOUND ( 'NONE', #206, .T. ) ;
#6104=FACE_OUTER_BOUND ( 'NONE', #2177, .T. ) ;
#6115=ADVANCED_FACE ( 'NONE', ( #4237 ), #433, .F. ) ;
#6120=CLOSED_SHELL ( 'NONE', ( #658, #6882, #6787, #5145, #6448, #399, #1620, #3326, #6060, #3040, #4483, #2882, #3141, #4997, #1242, #5801, #4617, #1333, #764, #6115, #3455, #890, #798, #2426, #1880, #4900, #704, #4555, #7590, #5912, #1104 ) ) ;
#6123=CARTESIAN_POINT ( 'NONE',  ( 119.9981648402866341, 207.8429183184022122, -120.0000000000000000 ) ) ;
#6127=EDGE_CURVE ( 'NONE', #4490, #746, #1444, .T. ) ;
#6129=VECTOR ( 'NONE', #1231, 1000.000000000000000 ) ;
#6140=DIRECTION ( 'NONE',  ( -0.000000000000000000, -0.000000000000000000, 1.000000000000000000 ) ) ;
#6142=PRODUCT_CONTEXT ( 'NONE', #567, 'mechanical' ) ;
#6146=ORIENTED_EDGE ( 'NONE', *, *, #3403, .T. ) ;
#6171=FACE_OUTER_BOUND ( 'NONE', #1650, .T. ) ;
#6172=CARTESIAN_POINT ( 'NONE',  ( 350.0000000000000000, -300.0000000000000000, -82.99999999999998579 ) ) ;
#6175=LINE ( 'NONE', #4389, #4558 ) ;
#6180=FACE_OUTER_BOUND ( 'NONE', #5931, .T. ) ;
#6181=DIRECTION ( 'NONE',  ( 1.000000000000000000, 0.000000000000000000, 0.000000000000000000 ) ) ;
#6195=ORIENTED_EDGE ( 'NONE', *, *, #6834, .T. ) ;
#6202=CIRCLE ( 'NONE', #2804, 5.250000000000004441 ) ;
#6205=CARTESIAN_POINT ( 'NONE',  ( 0.000000000000000000, 0.000000000000000000, -119.9999999999999858 ) ) ;
#6212=ORIENTED_EDGE ( 'NONE', *, *, #7331, .T. ) ;
#6215=VECTOR ( 'NONE', #1890, 1000.000000000000000 ) ;
#6220=DIRECTION ( 'NONE',  ( -0.000000000000000000, -0.000000000000000000, 1.000000000000000000 ) ) ;
#6260=DIRECTION ( 'NONE',  ( -0.000000000000000000, -0.000000000000000000, 1.000000000000000000 ) ) ;
#6264=EDGE_CURVE ( 'NONE', #1121, #6339, #6202, .T. ) ;
#6273=ORIENTED_EDGE ( 'NONE', *, *, #803, .T. ) ;
#6283=CARTESIAN_POINT ( 'NONE',  ( 279.9963296805736945, -6.714540835673234486E-12, -50.00000000000004263 ) ) ;
#6284=CARTESIAN_POINT ( 'NONE',  ( 37.49999999999997868, 0.000000000000000000, -90.00000000000000000 ) ) ;
#6288=VECTOR ( 'NONE', #957, 1000.000000000000000 ) ;
#6293=CYLINDRICAL_SURFACE ( 'NONE', #1364, 32.49999999999997158 ) ;
#6302=AXIS2_PLACEMENT_3D ( 'NONE', #5787, #7557, #4448 ) ;
#6305=EDGE_CURVE ( 'NONE', #1335, #6520, #6175, .T. ) ;
#6323=CYLINDRICAL_SURFACE ( 'NONE', #2726, 37.49999999999997868 ) ;
#6326=CARTESIAN_POINT ( 'NONE',  ( 207.8429183184021269, 119.9981648402868331, -120.0000000000000000 ) ) ;
#6339=VERTEX_POINT ( 'NONE', #5056 ) ;
#6359=EDGE_CURVE ( 'NONE', #1025, #1930, #4309, .T. ) ;
#6368=CARTESIAN_POINT ( 'NONE',  ( 350.0000000000000000, -300.0000000000000000, -120.0000000000000000 ) ) ;
#6377=EDGE_LOOP ( 'NONE', ( #2800, #4974, #2588, #5474 ) ) ;
#6381=CIRCLE ( 'NONE', #1855, 199.9963296805737230 ) ;
#6413=FACE_OUTER_BOUND ( 'NONE', #1779, .T. ) ;
#6414=CIRCLE ( 'NONE', #6041, 32.49999999999997158 ) ;
#6427=VERTEX_POINT ( 'NONE', #3768 ) ;
#6436=CARTESIAN_POINT ( 'NONE',  ( 0.000000000000000000, 0.000000000000000000, -112.9999999999999716 ) ) ;
#6438=VECTOR ( 'NONE', #4252, 1000.000000000000000 ) ;
#6441=ORIENTED_EDGE ( 'NONE', *, *, #4820, .T. ) ;
#6446=CARTESIAN_POINT ( 'NONE',  ( -199.9963296805737230, 2.449248649845333917E-14, 576.0908266162076643 ) ) ;
#6447=CARTESIAN_POINT ( 'NONE',  ( 202.5929183184021554, 119.9981648402868331, -120.0000000000000000 ) ) ;
#6448=ADVANCED_FACE ( 'NONE', ( #951 ), #4064, .F. ) ;
#6457=DIRECTION ( 'NONE',  ( 1.000000000000000000, 0.000000000000000000, 0.000000000000000000 ) ) ;
#6487=( GEOMETRIC_REPRESENTATION_CONTEXT ( 3 ) GLOBAL_UNCERTAINTY_ASSIGNED_CONTEXT ( ( #1374 ) ) GLOBAL_UNIT_ASSIGNED_CONTEXT ( ( #4771, #1858, #6744 ) ) REPRESENTATION_CONTEXT ( 'NONE', 'WORKASPACE' ) );
#6503=ORIENTED_EDGE ( 'NONE', *, *, #1138, .F. ) ;
#6505=ORIENTED_EDGE ( 'NONE', *, *, #4020, .F. ) ;
#6508=DIRECTION ( 'NONE',  ( 0.000000000000000000, 0.000000000000000000, -1.000000000000000000 ) ) ;
#6520=VERTEX_POINT ( 'NONE', #2190 ) ;
#6522=ORIENTED_EDGE ( 'NONE', *, *, #6127, .F. ) ;
#6550=DIRECTION ( 'NONE',  ( 1.000000000000000000, 0.000000000000000000, 0.000000000000000000 ) ) ;
#6551=AXIS2_PLACEMENT_3D ( 'NONE', #5660, #4134, #7216 ) ;
#6555=VECTOR ( 'NONE', #4101, 1000.000000000000000 ) ;
#6557=LINE ( 'NONE', #3435, #6555 ) ;
#6576=DIRECTION ( 'NONE',  ( -0.000000000000000000, -0.000000000000000000, -1.000000000000000000 ) ) ;
#6579=CARTESIAN_POINT ( 'NONE',  ( -350.0000000000000000, -299.9999999999998863, -82.99999999999998579 ) ) ;
#6584=ORIENTED_EDGE ( 'NONE', *, *, #1480, .F. ) ;
#6588=CIRCLE ( 'NONE', #3313, 5.250000000000004441 ) ;
#6608=DIRECTION ( 'NONE',  ( -1.000000000000000000, 1.586032892321652729E-16, 0.000000000000000000 ) ) ;
#6615=VERTEX_POINT ( 'NONE', #6007 ) ;
#6623=CARTESIAN_POINT ( 'NONE',  ( 202.5929183184021554, 119.9981648402868331, -50.00000000000000000 ) ) ;
#6631=ORIENTED_EDGE ( 'NONE', *, *, #4568, .T. ) ;
#6635=CIRCLE ( 'NONE', #833, 199.9963296805737230 ) ;
#6636=EDGE_CURVE ( 'NONE', #1540, #5426, #6588, .T. ) ;
#6658=FACE_BOUND ( 'NONE', #2451, .T. ) ;
#6661=EDGE_LOOP ( 'NONE', ( #5847, #6858, #6088, #2878 ) ) ;
#6663=AXIS2_PLACEMENT_3D ( 'NONE', #1885, #5396, #2994 ) ;
#6668=CIRCLE ( 'NONE', #6801, 37.49999999999997868 ) ;
#6671=CIRCLE ( 'NONE', #3779, 5.249999999999991118 ) ;
#6682=FACE_BOUND ( 'NONE', #5578, .T. ) ;
#6696=CARTESIAN_POINT ( 'NONE',  ( 0.000000000000000000, 0.000000000000000000, -82.99999999999998579 ) ) ;
#6699=ORIENTED_EDGE ( 'NONE', *, *, #5538, .T. ) ;
#6710=DIRECTION ( 'NONE',  ( 1.000000000000000000, 0.000000000000000000, 0.000000000000000000 ) ) ;
#6716=FACE_OUTER_BOUND ( 'NONE', #4150, .T. ) ;
#6720=CARTESIAN_POINT ( 'NONE',  ( -32.49999999999997158, 0.000000000000000000, -93.00430309513780003 ) ) ;
#6722=PRODUCT_DEFINITION ( 'UNKNOWN', '', #3064, #2364 ) ;
#6744=( NAMED_UNIT ( * ) SI_UNIT ( $, .STERADIAN. ) SOLID_ANGLE_UNIT ( ) );
#6755=VECTOR ( 'NONE', #3496, 1000.000000000000000 ) ;
#6756=DIRECTION ( 'NONE',  ( -0.000000000000000000, -0.000000000000000000, 1.000000000000000000 ) ) ;
#6763=DIRECTION ( 'NONE',  ( -0.000000000000000000, -0.000000000000000000, -1.000000000000000000 ) ) ;
#6774=DIRECTION ( 'NONE',  ( -1.000000000000000000, 0.000000000000000000, 0.000000000000000000 ) ) ;
#6778=PLANE ( 'NONE',  #1123 ) ;
#6787=ADVANCED_FACE ( 'NONE', ( #2544 ), #3205, .F. ) ;
#6800=ORIENTED_EDGE ( 'NONE', *, *, #5086, .F. ) ;
#6801=AXIS2_PLACEMENT_3D ( 'NONE', #2226, #2725, #4938 ) ;
#6802=DIRECTION ( 'NONE',  ( -1.000000000000000000, 0.000000000000000000, 0.000000000000000000 ) ) ;
#6808=DIRECTION ( 'NONE',  ( -0.000000000000000000, -0.000000000000000000, 1.000000000000000000 ) ) ;
#6812=FACE_OUTER_BOUND ( 'NONE', #3967, .T. ) ;
#6816=DIRECTION ( 'NONE',  ( 1.000000000000000000, 0.000000000000000000, 0.000000000000000000 ) ) ;
#6821=ORIENTED_EDGE ( 'NONE', *, *, #7219, .T. ) ;
#6825=DIRECTION ( 'NONE',  ( 1.000000000000000000, 0.000000000000000000, 0.000000000000000000 ) ) ;
#6834=EDGE_CURVE ( 'NONE', #6615, #7307, #7218, .T. ) ;
#6837=DIRECTION ( 'NONE',  ( 0.000000000000000000, 0.000000000000000000, 1.000000000000000000 ) ) ;
#6842=DIRECTION ( 'NONE',  ( -0.000000000000000000, -0.000000000000000000, 1.000000000000000000 ) ) ;
#6846=CIRCLE ( 'NONE', #2826, 37.49999999999997868 ) ;
#6853=CARTESIAN_POINT ( 'NONE',  ( 0.000000000000000000, 0.000000000000000000, -82.99999999999998579 ) ) ;
#6856=ORIENTED_EDGE ( 'NONE', *, *, #4071, .T. ) ;
#6858=ORIENTED_EDGE ( 'NONE', *, *, #6359, .F. ) ;
#6875=DIRECTION ( 'NONE',  ( 1.000000000000000000, 0.000000000000000000, 0.000000000000000000 ) ) ;
#6877=LINE ( 'NONE', #1391, #4119 ) ;
#6882=ADVANCED_FACE ( 'NONE', ( #7022 ), #6946, .F. ) ;
#6914=CARTESIAN_POINT ( 'NONE',  ( 114.7481648402866483, 207.8429183184022122, -50.00000000000000000 ) ) ;
#6922=VECTOR ( 'NONE', #4440, 1000.000000000000000 ) ;
#6935=DIRECTION ( 'NONE',  ( -1.000000000000000000, 0.000000000000000000, 0.000000000000000000 ) ) ;
#6942=VERTEX_POINT ( 'NONE', #5719 ) ;
#6946=CYLINDRICAL_SURFACE ( 'NONE', #3943, 5.249999999999976907 ) ;
#6947=ORIENTED_EDGE ( 'NONE', *, *, #6305, .T. ) ;
#6957=DIRECTION ( 'NONE',  ( -0.000000000000000000, -0.000000000000000000, 1.000000000000000000 ) ) ;
#6964=ORIENTED_EDGE ( 'NONE', *, *, #3261, .T. ) ;
#7005=ORIENTED_EDGE ( 'NONE', *, *, #470, .F. ) ;
#7011=DIRECTION ( 'NONE',  ( -0.000000000000000000, -0.000000000000000000, -1.000000000000000000 ) ) ;
#7021=DIRECTION ( 'NONE',  ( 1.000000000000000000, -1.224646799147352961E-16, 0.000000000000000000 ) ) ;
#7022=FACE_OUTER_BOUND ( 'NONE', #4256, .T. ) ;
#7037=FACE_OUTER_BOUND ( 'NONE', #5969, .T. ) ;
#7046=AXIS2_PLACEMENT_3D ( 'NONE', #1439, #6260, #847 ) ;
#7049=DIRECTION ( 'NONE',  ( 1.000000000000000000, 0.000000000000000000, 0.000000000000000000 ) ) ;
#7058=DIRECTION ( 'NONE',  ( -0.000000000000000000, -0.000000000000000000, 1.000000000000000000 ) ) ;
#7066=DIRECTION ( 'NONE',  ( 0.000000000000000000, 0.000000000000000000, 1.000000000000000000 ) ) ;
#7068=EDGE_CURVE ( 'NONE', #6427, #1238, #2490, .T. ) ;
#7069=EDGE_LOOP ( 'NONE', ( #4012, #3267 ) ) ;
#7070=EDGE_LOOP ( 'NONE', ( #3663, #7093, #6195, #2937 ) ) ;
#7082=EDGE_CURVE ( 'NONE', #4200, #2474, #2565, .T. ) ;
#7084=CARTESIAN_POINT ( 'NONE',  ( -202.5929183184026954, 119.9981648402859378, -120.0000000000000000 ) ) ;
#7093=ORIENTED_EDGE ( 'NONE', *, *, #5715, .T. ) ;
#7095=ORIENTED_EDGE ( 'NONE', *, *, #803, .F. ) ;
#7101=VECTOR ( 'NONE', #7058, 1000.000000000000000 ) ;
#7103=DIRECTION ( 'NONE',  ( -1.000000000000000000, 0.000000000000000000, 0.000000000000000000 ) ) ;
#7104=CARTESIAN_POINT ( 'NONE',  ( -5.134781488891348999E-13, 239.9963296805737230, -120.0000000000000000 ) ) ;
#7129=DIRECTION ( 'NONE',  ( -0.000000000000000000, -0.000000000000000000, 1.000000000000000000 ) ) ;
#7136=AXIS2_PLACEMENT_3D ( 'NONE', #4501, #3875, #6802 ) ;
#7146=CARTESIAN_POINT ( 'NONE',  ( -213.0929183184026670, 119.9981648402859378, -50.00000000000000000 ) ) ;
#7153=DIRECTION ( 'NONE',  ( -0.8571673007021121116, 1.049727191138618449E-16, 0.5150380749100544886 ) ) ;
#7184=EDGE_LOOP ( 'NONE', ( #3586, #5349, #3072, #2148 ) ) ;
#7187=EDGE_CURVE ( 'NONE', #1561, #1335, #376, .T. ) ;
#7188=CYLINDRICAL_SURFACE ( 'NONE', #3791, 37.49999999999997868 ) ;
#7198=FACE_BOUND ( 'NONE', #4743, .T. ) ;
#7202=ORIENTED_EDGE ( 'NONE', *, *, #7082, .F. ) ;
#7215=LINE ( 'NONE', #703, #4541 ) ;
#7216=DIRECTION ( 'NONE',  ( -1.000000000000000000, 0.000000000000000000, 0.000000000000000000 ) ) ;
#7218=CIRCLE ( 'NONE', #1934, 37.49999999999997868 ) ;
#7219=EDGE_CURVE ( 'NONE', #4399, #1948, #3969, .T. ) ;
#7236=CARTESIAN_POINT ( 'NONE',  ( 0.000000000000000000, 0.000000000000000000, -82.99999999999998579 ) ) ;
#7245=CARTESIAN_POINT ( 'NONE',  ( -5.250000000000505374, 239.9963296805737230, -50.00000000000000000 ) ) ;
#7246=DIRECTION ( 'NONE',  ( 1.000000000000000000, -1.586032892321652482E-16, 0.000000000000000000 ) ) ;
#7269=EDGE_CURVE ( 'NONE', #2058, #1947, #5152, .T. ) ;
#7273=CYLINDRICAL_SURFACE ( 'NONE', #7633, 5.249999999999976907 ) ;
#7275=DIRECTION ( 'NONE',  ( -1.000000000000000000, 0.000000000000000000, 0.000000000000000000 ) ) ;
#7281=CARTESIAN_POINT ( 'NONE',  ( -1.852913429037944315, 300.0000000000000568, -82.99999999999998579 ) ) ;
#7283=FACE_OUTER_BOUND ( 'NONE', #5701, .T. ) ;
#7292=ORIENTED_EDGE ( 'NONE', *, *, #5326, .T. ) ;
#7294=ORIENTED_EDGE ( 'NONE', *, *, #7310, .F. ) ;
#7297=PRESENTATION_STYLE_ASSIGNMENT (( #3 ) ) ;
#7307=VERTEX_POINT ( 'NONE', #1389 ) ;
#7310=EDGE_CURVE ( 'NONE', #2413, #1191, #3948, .T. ) ;
#7314=DIRECTION ( 'NONE',  ( -1.000000000000000000, 0.000000000000000000, 0.000000000000000000 ) ) ;
#7325=CARTESIAN_POINT ( 'NONE',  ( 125.2481648402866199, 207.8429183184022122, -120.0000000000000000 ) ) ;
#7331=EDGE_CURVE ( 'NONE', #1947, #7551, #6846, .T. ) ;
#7332=ORIENTED_EDGE ( 'NONE', *, *, #1677, .T. ) ;
#7361=DIRECTION ( 'NONE',  ( -0.000000000000000000, -0.000000000000000000, 1.000000000000000000 ) ) ;
#7363=AXIS2_PLACEMENT_3D ( 'NONE', #2124, #6957, #366 ) ;
#7365=DIRECTION ( 'NONE',  ( 1.000000000000000000, 0.000000000000000000, 0.000000000000000000 ) ) ;
#7370=CIRCLE ( 'NONE', #5218, 32.49999999999997158 ) ;
#7377=ORIENTED_EDGE ( 'NONE', *, *, #946, .T. ) ;
#7378=EDGE_LOOP ( 'NONE', ( #1221, #1590, #7332, #1757 ) ) ;
#7388=DIRECTION ( 'NONE',  ( 1.000000000000000000, 0.000000000000000000, 0.000000000000000000 ) ) ;
#7390=AXIS2_PLACEMENT_3D ( 'NONE', #2591, #4508, #1354 ) ;
#7413=VERTEX_POINT ( 'NONE', #6172 ) ;
#7423=CIRCLE ( 'NONE', #7046, 37.49999999999997868 ) ;
#7431=CARTESIAN_POINT ( 'NONE',  ( 0.000000000000000000, 0.000000000000000000, -82.99999999999998579 ) ) ;
#7433=DIRECTION ( 'NONE',  ( -0.000000000000000000, -0.000000000000000000, 1.000000000000000000 ) ) ;
#7437=DIRECTION ( 'NONE',  ( 1.000000000000000000, 0.000000000000000000, 0.000000000000000000 ) ) ;
#7439=ORIENTED_EDGE ( 'NONE', *, *, #1580, .F. ) ;
#7451=EDGE_CURVE ( 'NONE', #3050, #3424, #275, .T. ) ;
#7484=ORIENTED_EDGE ( 'NONE', *, *, #3028, .T. ) ;
#7485=AXIS2_PLACEMENT_3D ( 'NONE', #1301, #3758, #5977 ) ;
#7496=VECTOR ( 'NONE', #1432, 1000.000000000000000 ) ;
#7498=CARTESIAN_POINT ( 'NONE',  ( -207.8429183184026670, 119.9981648402859378, -50.00000000000000000 ) ) ;
#7521=ORIENTED_EDGE ( 'NONE', *, *, #5287, .F. ) ;
#7544=EDGE_CURVE ( 'NONE', #5402, #154, #5350, .T. ) ;
#7551=VERTEX_POINT ( 'NONE', #6284 ) ;
#7557=DIRECTION ( 'NONE',  ( -0.000000000000000000, -0.000000000000000000, -1.000000000000000000 ) ) ;
#7577=DIRECTION ( 'NONE',  ( -0.000000000000000000, -0.000000000000000000, 1.000000000000000000 ) ) ;
#7584=EDGE_CURVE ( 'NONE', #746, #1854, #3839, .T. ) ;
#7590=ADVANCED_FACE ( 'NONE', ( #7037 ), #7663, .F. ) ;
#7630=ORIENTED_EDGE ( 'NONE', *, *, #1372, .F. ) ;
#7633=AXIS2_PLACEMENT_3D ( 'NONE', #1873, #3136, #4267 ) ;
#7652=CARTESIAN_POINT ( 'NONE',  ( 213.0929183184020985, 119.9981648402868331, -120.0000000000000000 ) ) ;
#7661=DIRECTION ( 'NONE',  ( 1.000000000000000000, 0.000000000000000000, 0.000000000000000000 ) ) ;
#7663=CYLINDRICAL_SURFACE ( 'NONE', #7363, 5.249999999999992006 ) ;
#7665=DIRECTION ( 'NONE',  ( -0.000000000000000000, -0.000000000000000000, -1.000000000000000000 ) ) ;
#7667=DIRECTION ( 'NONE',  ( 0.000000000000000000, 0.000000000000000000, 1.000000000000000000 ) ) ;
#7677=LINE ( 'NONE', #6623, #2271 ) ;
#7686=DIRECTION ( 'NONE',  ( -1.000000000000000000, 1.224646799147352961E-16, 0.000000000000000000 ) ) ;
#7709=ORIENTED_EDGE ( 'NONE', *, *, #7584, .F. ) ;
#7710=EDGE_LOOP ( 'NONE', ( #2967, #899 ) ) ;
#7712=CARTESIAN_POINT ( 'NONE',  ( -5.134781488891348999E-13, 239.9963296805737230, -120.0000000000000000 ) ) ;
#7730=CIRCLE ( 'NONE', #4334, 5.249999999999995559 ) ;
#7747=EDGE_LOOP ( 'NONE', ( #2790, #7294 ) ) ;
#7748=ORIENTED_EDGE ( 'NONE', *, *, #3649, .F. ) ;
#7751=DIRECTION ( 'NONE',  ( 1.000000000000000000, 0.000000000000000000, 0.000000000000000000 ) ) ;
#7752=LINE ( 'NONE', #413, #4114 ) ;
#7803=COLOUR_RGB('Dark Blue',0.08,0.2,0.34);
#7804=FILL_AREA_STYLE_COLOUR('',#7803);
#7805=FILL_AREA_STYLE('',(#7804));
#7806=SURFACE_STYLE_FILL_AREA(#7805);
#7807=SURFACE_SIDE_STYLE('',(#7806));
#7808=SURFACE_STYLE_USAGE(.BOTH.,#7807);
#7809=PRESENTATION_STYLE_ASSIGNMENT((#7808));
ENDSEC;
END-ISO-10303-21;
